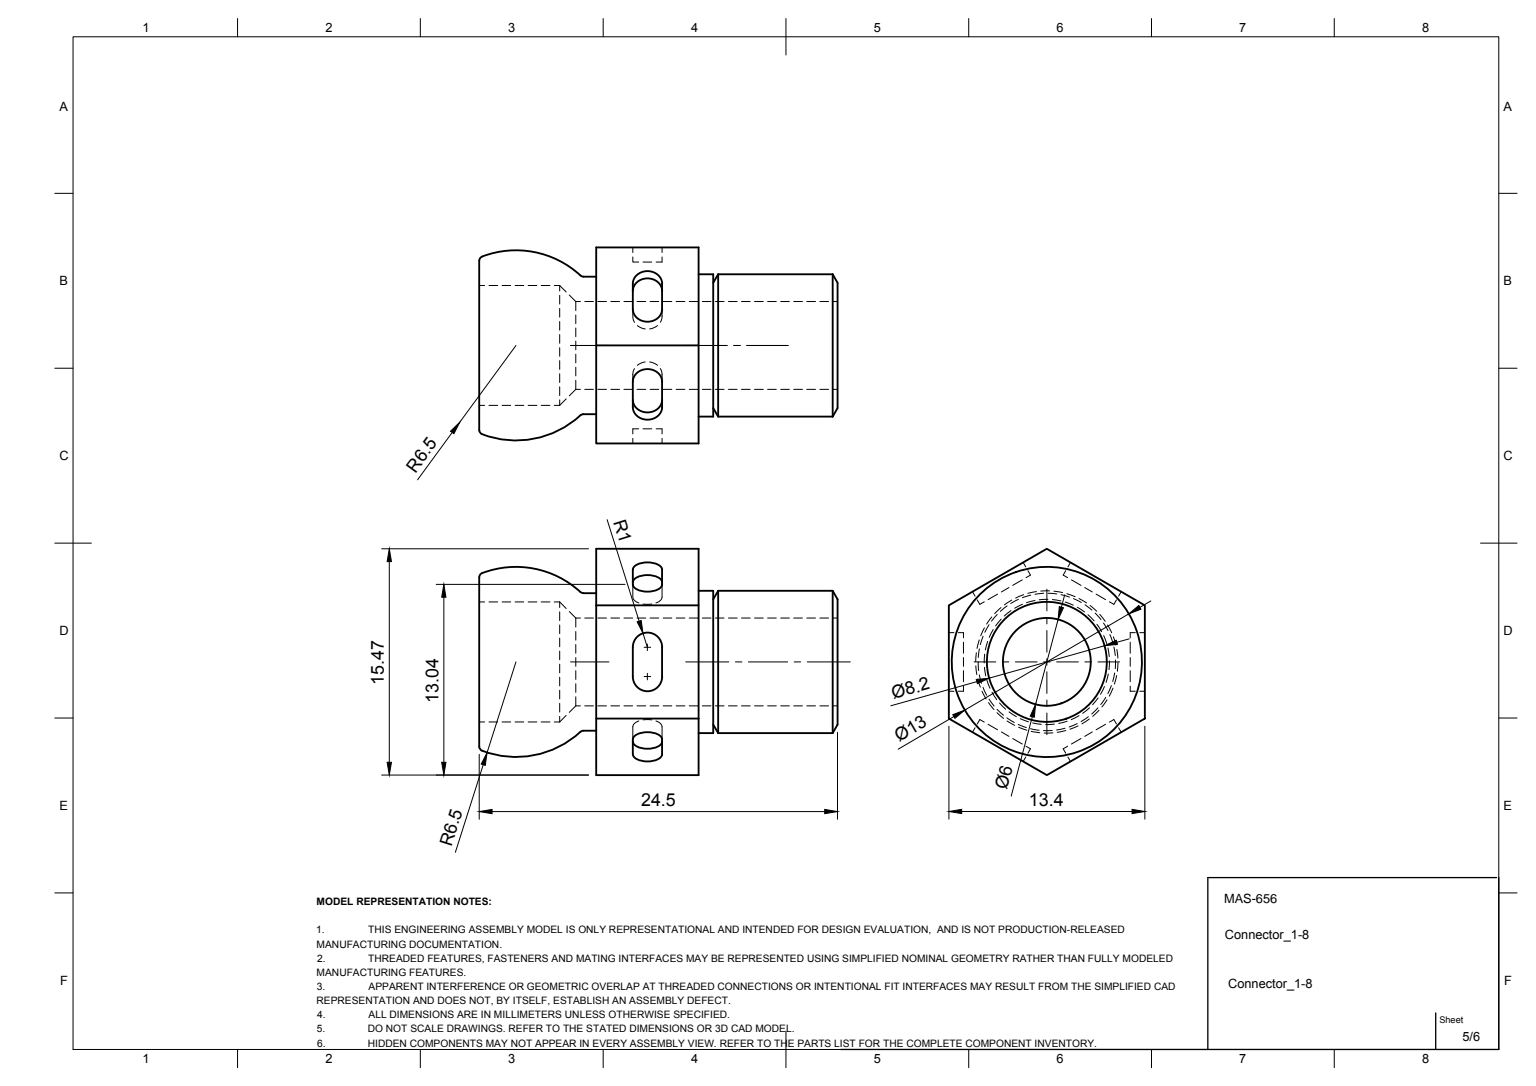
ISO-10303-21;
HEADER;
FILE_DESCRIPTION((''),'2;1');
FILE_NAME('Connector_1-8.step','2026-10-09T09:41:22-07:00',(''),(''),'','','');
FILE_SCHEMA (('AUTOMOTIVE_DESIGN { 1 0 10303 214 3 1 1 }'));
ENDSEC;
DATA;
#10=MECHANICAL_DESIGN_GEOMETRIC_PRESENTATION_REPRESENTATION('',(#74),#4304);
#66=SHAPE_REPRESENTATION_RELATIONSHIP('SRR','None',#4332,#70) ;
#70=ADVANCED_BREP_SHAPE_REPRESENTATION('',(#80),#4301) ;
#74=STYLED_ITEM('',(#4360),#80) ;
#80=MANIFOLD_SOLID_BREP('Body1',#2163) ;
#87=FACE_BOUND('',#638,.T.) ;
#88=FACE_BOUND('',#644,.T.) ;
#89=FACE_BOUND('',#648,.T.) ;
#90=FACE_BOUND('',#650,.T.) ;
#91=FACE_BOUND('',#652,.T.) ;
#92=FACE_BOUND('',#659,.T.) ;
#93=FACE_BOUND('',#661,.T.) ;
#94=FACE_BOUND('',#663,.T.) ;
#95=FACE_BOUND('',#665,.T.) ;
#96=FACE_BOUND('',#667,.T.) ;
#97=FACE_BOUND('',#694,.T.) ;
#119=PLANE('',#2272) ;
#120=PLANE('',#2282) ;
#121=PLANE('',#2288) ;
#122=PLANE('',#2289) ;
#123=PLANE('',#2291) ;
#124=PLANE('',#2296) ;
#125=PLANE('',#2297) ;
#126=PLANE('',#2298) ;
#127=PLANE('',#2301) ;
#128=PLANE('',#2304) ;
#129=PLANE('',#2307) ;
#130=PLANE('',#2310) ;
#131=PLANE('',#2313) ;
#132=PLANE('',#2318) ;
#133=PLANE('',#2319) ;
#134=PLANE('',#2320) ;
#135=PLANE('',#2325) ;
#136=PLANE('',#2326) ;
#137=PLANE('',#2327) ;
#138=PLANE('',#2332) ;
#139=PLANE('',#2333) ;
#140=PLANE('',#2334) ;
#141=PLANE('',#2339) ;
#142=PLANE('',#2340) ;
#143=PLANE('',#2341) ;
#144=PLANE('',#2346) ;
#145=PLANE('',#2347) ;
#146=PLANE('',#2348) ;
#147=PLANE('',#2351) ;
#167=TOROIDAL_SURFACE('',#2353,5.79274121460044,0.300000000000023) ;
#168=TOROIDAL_SURFACE('',#2364,5.00000000000038,0.300000000000023) ;
#181=CYLINDRICAL_SURFACE('',#2274,4.86400000000037) ;
#182=CYLINDRICAL_SURFACE('',#2276,3.00000000000023) ;
#183=CYLINDRICAL_SURFACE('',#2284,4.10000000000031) ;
#184=CYLINDRICAL_SURFACE('',#2286,4.86400000000037) ;
#185=CYLINDRICAL_SURFACE('',#2294,1.00000000000008) ;
#186=CYLINDRICAL_SURFACE('',#2300,1.00000000000008) ;
#187=CYLINDRICAL_SURFACE('',#2316,1.00000000000008) ;
#188=CYLINDRICAL_SURFACE('',#2322,1.00000000000008) ;
#189=CYLINDRICAL_SURFACE('',#2323,1.00000000000008) ;
#190=CYLINDRICAL_SURFACE('',#2329,1.00000000000008) ;
#191=CYLINDRICAL_SURFACE('',#2330,1.00000000000008) ;
#192=CYLINDRICAL_SURFACE('',#2336,1.00000000000008) ;
#193=CYLINDRICAL_SURFACE('',#2337,1.00000000000008) ;
#194=CYLINDRICAL_SURFACE('',#2343,1.00000000000008) ;
#195=CYLINDRICAL_SURFACE('',#2344,1.00000000000008) ;
#196=CYLINDRICAL_SURFACE('',#2350,1.00000000000008) ;
#197=CYLINDRICAL_SURFACE('',#2357,4.70000000000036) ;
#229=LINE('',#3374,#348) ;
#230=LINE('',#3382,#349) ;
#231=LINE('',#3385,#350) ;
#232=LINE('',#3389,#351) ;
#233=LINE('',#3393,#352) ;
#234=LINE('',#3400,#353) ;
#235=LINE('',#3405,#354) ;
#236=LINE('',#3409,#355) ;
#237=LINE('',#3411,#356) ;
#238=LINE('',#3413,#357) ;
#239=LINE('',#3415,#358) ;
#240=LINE('',#3417,#359) ;
#241=LINE('',#3418,#360) ;
#242=LINE('',#3422,#361) ;
#243=LINE('',#3424,#362) ;
#244=LINE('',#3426,#363) ;
#245=LINE('',#3428,#364) ;
#246=LINE('',#3430,#365) ;
#247=LINE('',#3431,#366) ;
#248=LINE('',#3435,#367) ;
#249=LINE('',#3436,#368) ;
#250=LINE('',#3441,#369) ;
#251=LINE('',#3444,#370) ;
#252=LINE('',#3447,#371) ;
#253=LINE('',#3449,#372) ;
#254=LINE('',#3453,#373) ;
#255=LINE('',#3454,#374) ;
#256=LINE('',#3457,#375) ;
#257=LINE('',#3458,#376) ;
#258=LINE('',#3463,#377) ;
#259=LINE('',#3466,#378) ;
#260=LINE('',#3470,#379) ;
#261=LINE('',#3473,#380) ;
#262=LINE('',#3476,#381) ;
#263=LINE('',#3480,#382) ;
#264=LINE('',#3483,#383) ;
#265=LINE('',#3486,#384) ;
#266=LINE('',#3490,#385) ;
#267=LINE('',#3493,#386) ;
#268=LINE('',#3496,#387) ;
#269=LINE('',#3500,#388) ;
#270=LINE('',#3505,#389) ;
#271=LINE('',#3509,#390) ;
#272=LINE('',#3513,#391) ;
#273=LINE('',#3515,#392) ;
#274=LINE('',#3519,#393) ;
#275=LINE('',#3520,#394) ;
#276=LINE('',#3523,#395) ;
#277=LINE('',#3524,#396) ;
#278=LINE('',#3530,#397) ;
#279=LINE('',#3532,#398) ;
#280=LINE('',#3536,#399) ;
#281=LINE('',#3537,#400) ;
#282=LINE('',#3540,#401) ;
#283=LINE('',#3541,#402) ;
#284=LINE('',#3547,#403) ;
#285=LINE('',#3549,#404) ;
#286=LINE('',#3553,#405) ;
#287=LINE('',#3554,#406) ;
#288=LINE('',#3557,#407) ;
#289=LINE('',#3558,#408) ;
#290=LINE('',#3564,#409) ;
#291=LINE('',#3566,#410) ;
#292=LINE('',#3570,#411) ;
#293=LINE('',#3571,#412) ;
#294=LINE('',#3574,#413) ;
#295=LINE('',#3575,#414) ;
#296=LINE('',#3581,#415) ;
#297=LINE('',#3583,#416) ;
#298=LINE('',#3587,#417) ;
#299=LINE('',#3588,#418) ;
#300=LINE('',#3591,#419) ;
#301=LINE('',#3592,#420) ;
#302=LINE('',#3609,#421) ;
#348=VECTOR('',#2652,4.28300000000033) ;
#349=VECTOR('',#2663,4.86400000000037) ;
#350=VECTOR('',#2666,3.00000000000023) ;
#351=VECTOR('',#2671,4.28300000000033) ;
#352=VECTOR('',#2676,3.00000000000023) ;
#353=VECTOR('',#2685,4.10000000000031) ;
#354=VECTOR('',#2692,4.86400000000037) ;
#355=VECTOR('',#2695,1.00000000000008) ;
#356=VECTOR('',#2696,0.999999999999697) ;
#357=VECTOR('',#2697,0.999999999999697) ;
#358=VECTOR('',#2698,1.00000000000008) ;
#359=VECTOR('',#2699,0.999999999999697) ;
#360=VECTOR('',#2700,0.999999999999697) ;
#361=VECTOR('',#2703,0.999999999999697) ;
#362=VECTOR('',#2704,1.00000000000008) ;
#363=VECTOR('',#2705,0.999999999999697) ;
#364=VECTOR('',#2706,0.999999999999697) ;
#365=VECTOR('',#2707,1.00000000000008) ;
#366=VECTOR('',#2708,0.999999999999697) ;
#367=VECTOR('',#2713,1.00000000000008) ;
#368=VECTOR('',#2714,1.00000000000008) ;
#369=VECTOR('',#2717,1.00000000000008) ;
#370=VECTOR('',#2720,1.00000000000008) ;
#371=VECTOR('',#2723,1.00000000000008) ;
#372=VECTOR('',#2724,1.00000000000008) ;
#373=VECTOR('',#2729,1.00000000000008) ;
#374=VECTOR('',#2730,1.00000000000008) ;
#375=VECTOR('',#2733,1.00000000000008) ;
#376=VECTOR('',#2734,1.00000000000008) ;
#377=VECTOR('',#2743,1.00000000000008) ;
#378=VECTOR('',#2744,0.999999999999697) ;
#379=VECTOR('',#2747,0.999999999999697) ;
#380=VECTOR('',#2752,1.00000000000008) ;
#381=VECTOR('',#2753,0.999999999999697) ;
#382=VECTOR('',#2756,0.999999999999697) ;
#383=VECTOR('',#2761,1.00000000000008) ;
#384=VECTOR('',#2762,0.999999999999697) ;
#385=VECTOR('',#2765,0.999999999999697) ;
#386=VECTOR('',#2770,1.00000000000008) ;
#387=VECTOR('',#2771,0.999999999999697) ;
#388=VECTOR('',#2774,0.999999999999697) ;
#389=VECTOR('',#2779,1.00000000000008) ;
#390=VECTOR('',#2782,1.00000000000008) ;
#391=VECTOR('',#2787,1.00000000000008) ;
#392=VECTOR('',#2788,1.00000000000008) ;
#393=VECTOR('',#2793,1.00000000000008) ;
#394=VECTOR('',#2794,1.00000000000008) ;
#395=VECTOR('',#2797,1.00000000000008) ;
#396=VECTOR('',#2798,1.00000000000008) ;
#397=VECTOR('',#2807,0.999999999999697) ;
#398=VECTOR('',#2808,0.999999999999697) ;
#399=VECTOR('',#2813,0.999999999999697) ;
#400=VECTOR('',#2814,0.999999999999697) ;
#401=VECTOR('',#2817,0.999999999999697) ;
#402=VECTOR('',#2818,0.999999999999697) ;
#403=VECTOR('',#2827,0.999999999999697) ;
#404=VECTOR('',#2828,0.999999999999697) ;
#405=VECTOR('',#2833,0.999999999999697) ;
#406=VECTOR('',#2834,0.999999999999697) ;
#407=VECTOR('',#2837,0.999999999999697) ;
#408=VECTOR('',#2838,0.999999999999697) ;
#409=VECTOR('',#2847,0.999999999999696) ;
#410=VECTOR('',#2848,0.999999999999696) ;
#411=VECTOR('',#2853,0.999999999999696) ;
#412=VECTOR('',#2854,0.999999999999697) ;
#413=VECTOR('',#2857,0.999999999999696) ;
#414=VECTOR('',#2858,0.999999999999697) ;
#415=VECTOR('',#2867,0.999999999999696) ;
#416=VECTOR('',#2868,0.999999999999696) ;
#417=VECTOR('',#2873,0.999999999999696) ;
#418=VECTOR('',#2874,0.999999999999697) ;
#419=VECTOR('',#2877,0.999999999999696) ;
#420=VECTOR('',#2878,0.999999999999697) ;
#421=VECTOR('',#2901,4.70000000000036) ;
#463=CONICAL_SURFACE('',#2269,4.28300000000033,1.0471975512) ;
#464=CONICAL_SURFACE('',#2278,4.28300000000033,1.0471975512) ;
#465=CONICAL_SURFACE('',#2280,3.00000000000023,0.785398163397) ;
#498=FACE_OUTER_BOUND('',#636,.T.) ;
#499=FACE_OUTER_BOUND('',#637,.T.) ;
#500=FACE_OUTER_BOUND('',#639,.T.) ;
#501=FACE_OUTER_BOUND('',#640,.T.) ;
#502=FACE_OUTER_BOUND('',#641,.T.) ;
#503=FACE_OUTER_BOUND('',#642,.T.) ;
#504=FACE_OUTER_BOUND('',#643,.T.) ;
#505=FACE_OUTER_BOUND('',#645,.T.) ;
#506=FACE_OUTER_BOUND('',#646,.T.) ;
#507=FACE_OUTER_BOUND('',#647,.T.) ;
#508=FACE_OUTER_BOUND('',#649,.T.) ;
#509=FACE_OUTER_BOUND('',#651,.T.) ;
#510=FACE_OUTER_BOUND('',#653,.T.) ;
#511=FACE_OUTER_BOUND('',#654,.T.) ;
#512=FACE_OUTER_BOUND('',#655,.T.) ;
#513=FACE_OUTER_BOUND('',#656,.T.) ;
#514=FACE_OUTER_BOUND('',#657,.T.) ;
#515=FACE_OUTER_BOUND('',#658,.T.) ;
#516=FACE_OUTER_BOUND('',#660,.T.) ;
#517=FACE_OUTER_BOUND('',#662,.T.) ;
#518=FACE_OUTER_BOUND('',#664,.T.) ;
#519=FACE_OUTER_BOUND('',#666,.T.) ;
#520=FACE_OUTER_BOUND('',#668,.T.) ;
#521=FACE_OUTER_BOUND('',#669,.T.) ;
#522=FACE_OUTER_BOUND('',#670,.T.) ;
#523=FACE_OUTER_BOUND('',#671,.T.) ;
#524=FACE_OUTER_BOUND('',#672,.T.) ;
#525=FACE_OUTER_BOUND('',#673,.T.) ;
#526=FACE_OUTER_BOUND('',#674,.T.) ;
#527=FACE_OUTER_BOUND('',#675,.T.) ;
#528=FACE_OUTER_BOUND('',#676,.T.) ;
#529=FACE_OUTER_BOUND('',#677,.T.) ;
#530=FACE_OUTER_BOUND('',#678,.T.) ;
#531=FACE_OUTER_BOUND('',#679,.T.) ;
#532=FACE_OUTER_BOUND('',#680,.T.) ;
#533=FACE_OUTER_BOUND('',#681,.T.) ;
#534=FACE_OUTER_BOUND('',#682,.T.) ;
#535=FACE_OUTER_BOUND('',#683,.T.) ;
#536=FACE_OUTER_BOUND('',#684,.T.) ;
#537=FACE_OUTER_BOUND('',#685,.T.) ;
#538=FACE_OUTER_BOUND('',#686,.T.) ;
#539=FACE_OUTER_BOUND('',#687,.T.) ;
#540=FACE_OUTER_BOUND('',#688,.T.) ;
#541=FACE_OUTER_BOUND('',#689,.T.) ;
#542=FACE_OUTER_BOUND('',#690,.T.) ;
#543=FACE_OUTER_BOUND('',#691,.T.) ;
#544=FACE_OUTER_BOUND('',#692,.T.) ;
#545=FACE_OUTER_BOUND('',#693,.T.) ;
#546=FACE_OUTER_BOUND('',#695,.T.) ;
#547=FACE_OUTER_BOUND('',#696,.T.) ;
#548=FACE_OUTER_BOUND('',#697,.T.) ;
#549=FACE_OUTER_BOUND('',#698,.T.) ;
#636=EDGE_LOOP('',(#1513,#1514,#1515,#1516)) ;
#637=EDGE_LOOP('',(#1517)) ;
#638=EDGE_LOOP('',(#1518)) ;
#639=EDGE_LOOP('',(#1519,#1520,#1521,#1522)) ;
#640=EDGE_LOOP('',(#1523,#1524,#1525,#1526)) ;
#641=EDGE_LOOP('',(#1527,#1528,#1529,#1530)) ;
#642=EDGE_LOOP('',(#1531,#1532,#1533,#1534)) ;
#643=EDGE_LOOP('',(#1535)) ;
#644=EDGE_LOOP('',(#1536)) ;
#645=EDGE_LOOP('',(#1537,#1538,#1539,#1540)) ;
#646=EDGE_LOOP('',(#1541,#1542,#1543,#1544)) ;
#647=EDGE_LOOP('',(#1545,#1546,#1547,#1548,#1549,#1550)) ;
#648=EDGE_LOOP('',(#1551)) ;
#649=EDGE_LOOP('',(#1552,#1553,#1554,#1555,#1556,#1557)) ;
#650=EDGE_LOOP('',(#1558)) ;
#651=EDGE_LOOP('',(#1559,#1560,#1561,#1562)) ;
#652=EDGE_LOOP('',(#1563,#1564,#1565,#1566)) ;
#653=EDGE_LOOP('',(#1567,#1568,#1569,#1570)) ;
#654=EDGE_LOOP('',(#1571,#1572,#1573,#1574)) ;
#655=EDGE_LOOP('',(#1575,#1576,#1577,#1578)) ;
#656=EDGE_LOOP('',(#1579,#1580,#1581,#1582)) ;
#657=EDGE_LOOP('',(#1583,#1584,#1585,#1586)) ;
#658=EDGE_LOOP('',(#1587,#1588,#1589,#1590)) ;
#659=EDGE_LOOP('',(#1591,#1592,#1593,#1594)) ;
#660=EDGE_LOOP('',(#1595,#1596,#1597,#1598)) ;
#661=EDGE_LOOP('',(#1599,#1600,#1601,#1602)) ;
#662=EDGE_LOOP('',(#1603,#1604,#1605,#1606)) ;
#663=EDGE_LOOP('',(#1607,#1608,#1609,#1610)) ;
#664=EDGE_LOOP('',(#1611,#1612,#1613,#1614)) ;
#665=EDGE_LOOP('',(#1615,#1616,#1617,#1618)) ;
#666=EDGE_LOOP('',(#1619,#1620,#1621,#1622)) ;
#667=EDGE_LOOP('',(#1623,#1624,#1625,#1626)) ;
#668=EDGE_LOOP('',(#1627,#1628,#1629,#1630)) ;
#669=EDGE_LOOP('',(#1631,#1632,#1633,#1634)) ;
#670=EDGE_LOOP('',(#1635,#1636,#1637,#1638)) ;
#671=EDGE_LOOP('',(#1639,#1640,#1641,#1642)) ;
#672=EDGE_LOOP('',(#1643,#1644,#1645,#1646)) ;
#673=EDGE_LOOP('',(#1647,#1648,#1649,#1650)) ;
#674=EDGE_LOOP('',(#1651,#1652,#1653,#1654)) ;
#675=EDGE_LOOP('',(#1655,#1656,#1657,#1658)) ;
#676=EDGE_LOOP('',(#1659,#1660,#1661,#1662)) ;
#677=EDGE_LOOP('',(#1663,#1664,#1665,#1666)) ;
#678=EDGE_LOOP('',(#1667,#1668,#1669,#1670)) ;
#679=EDGE_LOOP('',(#1671,#1672,#1673,#1674)) ;
#680=EDGE_LOOP('',(#1675,#1676,#1677,#1678)) ;
#681=EDGE_LOOP('',(#1679,#1680,#1681,#1682)) ;
#682=EDGE_LOOP('',(#1683,#1684,#1685,#1686)) ;
#683=EDGE_LOOP('',(#1687,#1688,#1689,#1690)) ;
#684=EDGE_LOOP('',(#1691,#1692,#1693,#1694)) ;
#685=EDGE_LOOP('',(#1695,#1696,#1697,#1698)) ;
#686=EDGE_LOOP('',(#1699,#1700,#1701,#1702)) ;
#687=EDGE_LOOP('',(#1703,#1704,#1705,#1706)) ;
#688=EDGE_LOOP('',(#1707,#1708,#1709,#1710)) ;
#689=EDGE_LOOP('',(#1711,#1712,#1713,#1714)) ;
#690=EDGE_LOOP('',(#1715,#1716,#1717,#1718)) ;
#691=EDGE_LOOP('',(#1719,#1720,#1721,#1722)) ;
#692=EDGE_LOOP('',(#1723,#1724,#1725,#1726)) ;
#693=EDGE_LOOP('',(#1727)) ;
#694=EDGE_LOOP('',(#1728)) ;
#695=EDGE_LOOP('',(#1729,#1730,#1731,#1732,#1733)) ;
#696=EDGE_LOOP('',(#1734,#1735,#1736,#1737,#1738)) ;
#697=EDGE_LOOP('',(#1739,#1740,#1741,#1742,#1743,#1744)) ;
#698=EDGE_LOOP('',(#1745,#1746,#1747,#1748,#1749,#1750)) ;
#819=CIRCLE('',#2270,4.86400000000037) ;
#820=CIRCLE('',#2271,4.28300000000033) ;
#821=CIRCLE('',#2273,3.00000000000023) ;
#822=CIRCLE('',#2275,4.86400000000037) ;
#823=CIRCLE('',#2277,3.00000000000023) ;
#824=CIRCLE('',#2279,4.28300000000033) ;
#825=CIRCLE('',#2281,4.10000000000031) ;
#826=CIRCLE('',#2283,4.86400000000037) ;
#827=CIRCLE('',#2285,4.10000000000031) ;
#828=CIRCLE('',#2287,4.86400000000037) ;
#829=CIRCLE('',#2290,4.70000000000036) ;
#830=CIRCLE('',#2292,1.00000000000008) ;
#831=CIRCLE('',#2293,1.00000000000008) ;
#832=CIRCLE('',#2295,1.00000000000008) ;
#833=CIRCLE('',#2299,1.00000000000008) ;
#834=CIRCLE('',#2302,1.00000000000008) ;
#835=CIRCLE('',#2303,1.00000000000008) ;
#836=CIRCLE('',#2305,1.00000000000008) ;
#837=CIRCLE('',#2306,1.00000000000008) ;
#838=CIRCLE('',#2308,1.00000000000008) ;
#839=CIRCLE('',#2309,1.00000000000008) ;
#840=CIRCLE('',#2311,1.00000000000008) ;
#841=CIRCLE('',#2312,1.00000000000008) ;
#842=CIRCLE('',#2314,1.00000000000008) ;
#843=CIRCLE('',#2315,1.00000000000008) ;
#844=CIRCLE('',#2317,1.00000000000008) ;
#845=CIRCLE('',#2321,1.00000000000008) ;
#846=CIRCLE('',#2324,1.00000000000008) ;
#847=CIRCLE('',#2328,1.00000000000008) ;
#848=CIRCLE('',#2331,1.00000000000008) ;
#849=CIRCLE('',#2335,1.00000000000008) ;
#850=CIRCLE('',#2338,1.00000000000008) ;
#851=CIRCLE('',#2342,1.00000000000008) ;
#852=CIRCLE('',#2345,1.00000000000008) ;
#853=CIRCLE('',#2349,1.00000000000008) ;
#854=CIRCLE('',#2352,5.79274121460045) ;
#855=CIRCLE('',#2354,0.300000000000023) ;
#856=CIRCLE('',#2355,6.07303514434047) ;
#857=CIRCLE('',#2356,6.07303514434047) ;
#858=CIRCLE('',#2358,4.70000000000036) ;
#859=CIRCLE('',#2359,4.70000000000036) ;
#860=CIRCLE('',#2361,6.50000000000051) ;
#861=CIRCLE('',#2362,4.77941176471037) ;
#862=CIRCLE('',#2363,4.77941176471037) ;
#863=CIRCLE('',#2365,0.300000000000023) ;
#978=VERTEX_POINT('',#3371) ;
#979=VERTEX_POINT('',#3373) ;
#980=VERTEX_POINT('',#3377) ;
#981=VERTEX_POINT('',#3380) ;
#982=VERTEX_POINT('',#3384) ;
#983=VERTEX_POINT('',#3388) ;
#984=VERTEX_POINT('',#3392) ;
#985=VERTEX_POINT('',#3396) ;
#986=VERTEX_POINT('',#3399) ;
#987=VERTEX_POINT('',#3403) ;
#988=VERTEX_POINT('',#3407) ;
#989=VERTEX_POINT('',#3408) ;
#990=VERTEX_POINT('',#3410) ;
#991=VERTEX_POINT('',#3412) ;
#992=VERTEX_POINT('',#3414) ;
#993=VERTEX_POINT('',#3416) ;
#994=VERTEX_POINT('',#3420) ;
#995=VERTEX_POINT('',#3421) ;
#996=VERTEX_POINT('',#3423) ;
#997=VERTEX_POINT('',#3425) ;
#998=VERTEX_POINT('',#3427) ;
#999=VERTEX_POINT('',#3429) ;
#1000=VERTEX_POINT('',#3432) ;
#1001=VERTEX_POINT('',#3437) ;
#1002=VERTEX_POINT('',#3438) ;
#1003=VERTEX_POINT('',#3440) ;
#1004=VERTEX_POINT('',#3442) ;
#1005=VERTEX_POINT('',#3446) ;
#1006=VERTEX_POINT('',#3448) ;
#1007=VERTEX_POINT('',#3452) ;
#1008=VERTEX_POINT('',#3456) ;
#1009=VERTEX_POINT('',#3464) ;
#1010=VERTEX_POINT('',#3465) ;
#1011=VERTEX_POINT('',#3467) ;
#1012=VERTEX_POINT('',#3469) ;
#1013=VERTEX_POINT('',#3474) ;
#1014=VERTEX_POINT('',#3475) ;
#1015=VERTEX_POINT('',#3477) ;
#1016=VERTEX_POINT('',#3479) ;
#1017=VERTEX_POINT('',#3484) ;
#1018=VERTEX_POINT('',#3485) ;
#1019=VERTEX_POINT('',#3487) ;
#1020=VERTEX_POINT('',#3489) ;
#1021=VERTEX_POINT('',#3494) ;
#1022=VERTEX_POINT('',#3495) ;
#1023=VERTEX_POINT('',#3497) ;
#1024=VERTEX_POINT('',#3499) ;
#1025=VERTEX_POINT('',#3503) ;
#1026=VERTEX_POINT('',#3504) ;
#1027=VERTEX_POINT('',#3506) ;
#1028=VERTEX_POINT('',#3508) ;
#1029=VERTEX_POINT('',#3512) ;
#1030=VERTEX_POINT('',#3514) ;
#1031=VERTEX_POINT('',#3518) ;
#1032=VERTEX_POINT('',#3522) ;
#1033=VERTEX_POINT('',#3529) ;
#1034=VERTEX_POINT('',#3531) ;
#1035=VERTEX_POINT('',#3535) ;
#1036=VERTEX_POINT('',#3539) ;
#1037=VERTEX_POINT('',#3546) ;
#1038=VERTEX_POINT('',#3548) ;
#1039=VERTEX_POINT('',#3552) ;
#1040=VERTEX_POINT('',#3556) ;
#1041=VERTEX_POINT('',#3563) ;
#1042=VERTEX_POINT('',#3565) ;
#1043=VERTEX_POINT('',#3569) ;
#1044=VERTEX_POINT('',#3573) ;
#1045=VERTEX_POINT('',#3580) ;
#1046=VERTEX_POINT('',#3582) ;
#1047=VERTEX_POINT('',#3586) ;
#1048=VERTEX_POINT('',#3590) ;
#1049=VERTEX_POINT('',#3597) ;
#1050=VERTEX_POINT('',#3600) ;
#1051=VERTEX_POINT('',#3602) ;
#1052=VERTEX_POINT('',#3606) ;
#1053=VERTEX_POINT('',#3607) ;
#1054=VERTEX_POINT('',#3612) ;
#1055=VERTEX_POINT('',#3614) ;
#1178=EDGE_CURVE('',#978,#978,#819,.T.) ;
#1179=EDGE_CURVE('',#978,#979,#229,.T.) ;
#1180=EDGE_CURVE('',#979,#979,#820,.T.) ;
#1181=EDGE_CURVE('',#980,#980,#821,.T.) ;
#1182=EDGE_CURVE('',#981,#981,#822,.T.) ;
#1183=EDGE_CURVE('',#981,#978,#230,.T.) ;
#1184=EDGE_CURVE('',#980,#982,#231,.T.) ;
#1185=EDGE_CURVE('',#982,#982,#823,.T.) ;
#1186=EDGE_CURVE('',#981,#983,#232,.T.) ;
#1187=EDGE_CURVE('',#983,#983,#824,.F.) ;
#1188=EDGE_CURVE('',#982,#984,#233,.T.) ;
#1189=EDGE_CURVE('',#984,#984,#825,.T.) ;
#1190=EDGE_CURVE('',#985,#985,#826,.T.) ;
#1191=EDGE_CURVE('',#984,#986,#234,.T.) ;
#1192=EDGE_CURVE('',#986,#986,#827,.T.) ;
#1193=EDGE_CURVE('',#987,#987,#828,.T.) ;
#1194=EDGE_CURVE('',#987,#985,#235,.T.) ;
#1195=EDGE_CURVE('',#988,#989,#236,.T.) ;
#1196=EDGE_CURVE('',#989,#990,#237,.T.) ;
#1197=EDGE_CURVE('',#990,#991,#238,.T.) ;
#1198=EDGE_CURVE('',#991,#992,#239,.T.) ;
#1199=EDGE_CURVE('',#992,#993,#240,.T.) ;
#1200=EDGE_CURVE('',#993,#988,#241,.T.) ;
#1201=EDGE_CURVE('',#994,#995,#242,.T.) ;
#1202=EDGE_CURVE('',#996,#994,#243,.T.) ;
#1203=EDGE_CURVE('',#997,#996,#244,.T.) ;
#1204=EDGE_CURVE('',#998,#997,#245,.T.) ;
#1205=EDGE_CURVE('',#999,#998,#246,.T.) ;
#1206=EDGE_CURVE('',#995,#999,#247,.T.) ;
#1207=EDGE_CURVE('',#1000,#1000,#829,.T.) ;
#1208=EDGE_CURVE('',#992,#994,#248,.T.) ;
#1209=EDGE_CURVE('',#991,#996,#249,.T.) ;
#1210=EDGE_CURVE('',#1001,#1002,#830,.F.) ;
#1211=EDGE_CURVE('',#1003,#1001,#250,.F.) ;
#1212=EDGE_CURVE('',#1004,#1003,#831,.F.) ;
#1213=EDGE_CURVE('',#1002,#1004,#251,.F.) ;
#1214=EDGE_CURVE('',#1004,#1005,#252,.F.) ;
#1215=EDGE_CURVE('',#1003,#1006,#253,.F.) ;
#1216=EDGE_CURVE('',#1005,#1006,#832,.T.) ;
#1217=EDGE_CURVE('',#1002,#1007,#254,.T.) ;
#1218=EDGE_CURVE('',#1007,#1005,#255,.F.) ;
#1219=EDGE_CURVE('',#1001,#1008,#256,.T.) ;
#1220=EDGE_CURVE('',#1006,#1008,#257,.F.) ;
#1221=EDGE_CURVE('',#1008,#1007,#833,.T.) ;
#1222=EDGE_CURVE('',#990,#997,#258,.T.) ;
#1223=EDGE_CURVE('',#1009,#1010,#259,.F.) ;
#1224=EDGE_CURVE('',#1011,#1009,#834,.F.) ;
#1225=EDGE_CURVE('',#1012,#1011,#260,.F.) ;
#1226=EDGE_CURVE('',#1010,#1012,#835,.F.) ;
#1227=EDGE_CURVE('',#993,#995,#261,.T.) ;
#1228=EDGE_CURVE('',#1013,#1014,#262,.F.) ;
#1229=EDGE_CURVE('',#1015,#1013,#836,.F.) ;
#1230=EDGE_CURVE('',#1016,#1015,#263,.F.) ;
#1231=EDGE_CURVE('',#1014,#1016,#837,.F.) ;
#1232=EDGE_CURVE('',#989,#998,#264,.T.) ;
#1233=EDGE_CURVE('',#1017,#1018,#265,.F.) ;
#1234=EDGE_CURVE('',#1019,#1017,#838,.F.) ;
#1235=EDGE_CURVE('',#1020,#1019,#266,.F.) ;
#1236=EDGE_CURVE('',#1018,#1020,#839,.F.) ;
#1237=EDGE_CURVE('',#988,#999,#267,.T.) ;
#1238=EDGE_CURVE('',#1021,#1022,#268,.F.) ;
#1239=EDGE_CURVE('',#1023,#1021,#840,.F.) ;
#1240=EDGE_CURVE('',#1024,#1023,#269,.F.) ;
#1241=EDGE_CURVE('',#1022,#1024,#841,.F.) ;
#1242=EDGE_CURVE('',#1025,#1026,#270,.F.) ;
#1243=EDGE_CURVE('',#1027,#1025,#842,.F.) ;
#1244=EDGE_CURVE('',#1028,#1027,#271,.F.) ;
#1245=EDGE_CURVE('',#1026,#1028,#843,.F.) ;
#1246=EDGE_CURVE('',#1027,#1029,#272,.F.) ;
#1247=EDGE_CURVE('',#1025,#1030,#273,.F.) ;
#1248=EDGE_CURVE('',#1029,#1030,#844,.T.) ;
#1249=EDGE_CURVE('',#1028,#1031,#274,.T.) ;
#1250=EDGE_CURVE('',#1031,#1029,#275,.F.) ;
#1251=EDGE_CURVE('',#1026,#1032,#276,.T.) ;
#1252=EDGE_CURVE('',#1030,#1032,#277,.F.) ;
#1253=EDGE_CURVE('',#1032,#1031,#845,.T.) ;
#1254=EDGE_CURVE('',#1015,#1033,#278,.F.) ;
#1255=EDGE_CURVE('',#1013,#1034,#279,.F.) ;
#1256=EDGE_CURVE('',#1033,#1034,#846,.T.) ;
#1257=EDGE_CURVE('',#1016,#1035,#280,.T.) ;
#1258=EDGE_CURVE('',#1035,#1033,#281,.F.) ;
#1259=EDGE_CURVE('',#1014,#1036,#282,.T.) ;
#1260=EDGE_CURVE('',#1034,#1036,#283,.F.) ;
#1261=EDGE_CURVE('',#1036,#1035,#847,.T.) ;
#1262=EDGE_CURVE('',#1019,#1037,#284,.F.) ;
#1263=EDGE_CURVE('',#1017,#1038,#285,.F.) ;
#1264=EDGE_CURVE('',#1037,#1038,#848,.T.) ;
#1265=EDGE_CURVE('',#1020,#1039,#286,.T.) ;
#1266=EDGE_CURVE('',#1039,#1037,#287,.F.) ;
#1267=EDGE_CURVE('',#1018,#1040,#288,.T.) ;
#1268=EDGE_CURVE('',#1038,#1040,#289,.F.) ;
#1269=EDGE_CURVE('',#1040,#1039,#849,.T.) ;
#1270=EDGE_CURVE('',#1011,#1041,#290,.F.) ;
#1271=EDGE_CURVE('',#1009,#1042,#291,.F.) ;
#1272=EDGE_CURVE('',#1041,#1042,#850,.T.) ;
#1273=EDGE_CURVE('',#1012,#1043,#292,.T.) ;
#1274=EDGE_CURVE('',#1043,#1041,#293,.F.) ;
#1275=EDGE_CURVE('',#1010,#1044,#294,.T.) ;
#1276=EDGE_CURVE('',#1042,#1044,#295,.F.) ;
#1277=EDGE_CURVE('',#1044,#1043,#851,.T.) ;
#1278=EDGE_CURVE('',#1023,#1045,#296,.F.) ;
#1279=EDGE_CURVE('',#1021,#1046,#297,.F.) ;
#1280=EDGE_CURVE('',#1045,#1046,#852,.T.) ;
#1281=EDGE_CURVE('',#1024,#1047,#298,.T.) ;
#1282=EDGE_CURVE('',#1047,#1045,#299,.F.) ;
#1283=EDGE_CURVE('',#1022,#1048,#300,.T.) ;
#1284=EDGE_CURVE('',#1046,#1048,#301,.F.) ;
#1285=EDGE_CURVE('',#1048,#1047,#853,.T.) ;
#1286=EDGE_CURVE('',#1049,#1049,#854,.T.) ;
#1287=EDGE_CURVE('',#1049,#1050,#855,.T.) ;
#1288=EDGE_CURVE('',#1050,#1051,#856,.T.) ;
#1289=EDGE_CURVE('',#1051,#1050,#857,.T.) ;
#1290=EDGE_CURVE('',#1052,#1053,#858,.F.) ;
#1291=EDGE_CURVE('',#1053,#1000,#302,.T.) ;
#1292=EDGE_CURVE('',#1053,#1052,#859,.F.) ;
#1293=EDGE_CURVE('',#1051,#1054,#860,.T.) ;
#1294=EDGE_CURVE('',#1055,#1054,#861,.F.) ;
#1295=EDGE_CURVE('',#1054,#1055,#862,.F.) ;
#1296=EDGE_CURVE('',#1055,#1052,#863,.T.) ;
#1513=ORIENTED_EDGE('',*,*,#1178,.F.) ;
#1514=ORIENTED_EDGE('',*,*,#1179,.T.) ;
#1515=ORIENTED_EDGE('',*,*,#1180,.T.) ;
#1516=ORIENTED_EDGE('',*,*,#1179,.F.) ;
#1517=ORIENTED_EDGE('',*,*,#1180,.F.) ;
#1518=ORIENTED_EDGE('',*,*,#1181,.T.) ;
#1519=ORIENTED_EDGE('',*,*,#1182,.F.) ;
#1520=ORIENTED_EDGE('',*,*,#1183,.T.) ;
#1521=ORIENTED_EDGE('',*,*,#1178,.T.) ;
#1522=ORIENTED_EDGE('',*,*,#1183,.F.) ;
#1523=ORIENTED_EDGE('',*,*,#1181,.F.) ;
#1524=ORIENTED_EDGE('',*,*,#1184,.T.) ;
#1525=ORIENTED_EDGE('',*,*,#1185,.T.) ;
#1526=ORIENTED_EDGE('',*,*,#1184,.F.) ;
#1527=ORIENTED_EDGE('',*,*,#1182,.T.) ;
#1528=ORIENTED_EDGE('',*,*,#1186,.T.) ;
#1529=ORIENTED_EDGE('',*,*,#1187,.F.) ;
#1530=ORIENTED_EDGE('',*,*,#1186,.F.) ;
#1531=ORIENTED_EDGE('',*,*,#1185,.F.) ;
#1532=ORIENTED_EDGE('',*,*,#1188,.T.) ;
#1533=ORIENTED_EDGE('',*,*,#1189,.T.) ;
#1534=ORIENTED_EDGE('',*,*,#1188,.F.) ;
#1535=ORIENTED_EDGE('',*,*,#1190,.F.) ;
#1536=ORIENTED_EDGE('',*,*,#1187,.T.) ;
#1537=ORIENTED_EDGE('',*,*,#1189,.F.) ;
#1538=ORIENTED_EDGE('',*,*,#1191,.T.) ;
#1539=ORIENTED_EDGE('',*,*,#1192,.T.) ;
#1540=ORIENTED_EDGE('',*,*,#1191,.F.) ;
#1541=ORIENTED_EDGE('',*,*,#1193,.F.) ;
#1542=ORIENTED_EDGE('',*,*,#1194,.T.) ;
#1543=ORIENTED_EDGE('',*,*,#1190,.T.) ;
#1544=ORIENTED_EDGE('',*,*,#1194,.F.) ;
#1545=ORIENTED_EDGE('',*,*,#1195,.T.) ;
#1546=ORIENTED_EDGE('',*,*,#1196,.T.) ;
#1547=ORIENTED_EDGE('',*,*,#1197,.T.) ;
#1548=ORIENTED_EDGE('',*,*,#1198,.T.) ;
#1549=ORIENTED_EDGE('',*,*,#1199,.T.) ;
#1550=ORIENTED_EDGE('',*,*,#1200,.T.) ;
#1551=ORIENTED_EDGE('',*,*,#1193,.T.) ;
#1552=ORIENTED_EDGE('',*,*,#1201,.F.) ;
#1553=ORIENTED_EDGE('',*,*,#1202,.F.) ;
#1554=ORIENTED_EDGE('',*,*,#1203,.F.) ;
#1555=ORIENTED_EDGE('',*,*,#1204,.F.) ;
#1556=ORIENTED_EDGE('',*,*,#1205,.F.) ;
#1557=ORIENTED_EDGE('',*,*,#1206,.F.) ;
#1558=ORIENTED_EDGE('',*,*,#1207,.F.) ;
#1559=ORIENTED_EDGE('',*,*,#1202,.T.) ;
#1560=ORIENTED_EDGE('',*,*,#1208,.F.) ;
#1561=ORIENTED_EDGE('',*,*,#1198,.F.) ;
#1562=ORIENTED_EDGE('',*,*,#1209,.T.) ;
#1563=ORIENTED_EDGE('',*,*,#1210,.F.) ;
#1564=ORIENTED_EDGE('',*,*,#1211,.F.) ;
#1565=ORIENTED_EDGE('',*,*,#1212,.F.) ;
#1566=ORIENTED_EDGE('',*,*,#1213,.F.) ;
#1567=ORIENTED_EDGE('',*,*,#1214,.F.) ;
#1568=ORIENTED_EDGE('',*,*,#1212,.T.) ;
#1569=ORIENTED_EDGE('',*,*,#1215,.T.) ;
#1570=ORIENTED_EDGE('',*,*,#1216,.F.) ;
#1571=ORIENTED_EDGE('',*,*,#1217,.F.) ;
#1572=ORIENTED_EDGE('',*,*,#1213,.T.) ;
#1573=ORIENTED_EDGE('',*,*,#1214,.T.) ;
#1574=ORIENTED_EDGE('',*,*,#1218,.F.) ;
#1575=ORIENTED_EDGE('',*,*,#1215,.F.) ;
#1576=ORIENTED_EDGE('',*,*,#1211,.T.) ;
#1577=ORIENTED_EDGE('',*,*,#1219,.T.) ;
#1578=ORIENTED_EDGE('',*,*,#1220,.F.) ;
#1579=ORIENTED_EDGE('',*,*,#1216,.T.) ;
#1580=ORIENTED_EDGE('',*,*,#1220,.T.) ;
#1581=ORIENTED_EDGE('',*,*,#1221,.T.) ;
#1582=ORIENTED_EDGE('',*,*,#1218,.T.) ;
#1583=ORIENTED_EDGE('',*,*,#1219,.F.) ;
#1584=ORIENTED_EDGE('',*,*,#1210,.T.) ;
#1585=ORIENTED_EDGE('',*,*,#1217,.T.) ;
#1586=ORIENTED_EDGE('',*,*,#1221,.F.) ;
#1587=ORIENTED_EDGE('',*,*,#1203,.T.) ;
#1588=ORIENTED_EDGE('',*,*,#1209,.F.) ;
#1589=ORIENTED_EDGE('',*,*,#1197,.F.) ;
#1590=ORIENTED_EDGE('',*,*,#1222,.T.) ;
#1591=ORIENTED_EDGE('',*,*,#1223,.F.) ;
#1592=ORIENTED_EDGE('',*,*,#1224,.F.) ;
#1593=ORIENTED_EDGE('',*,*,#1225,.F.) ;
#1594=ORIENTED_EDGE('',*,*,#1226,.F.) ;
#1595=ORIENTED_EDGE('',*,*,#1201,.T.) ;
#1596=ORIENTED_EDGE('',*,*,#1227,.F.) ;
#1597=ORIENTED_EDGE('',*,*,#1199,.F.) ;
#1598=ORIENTED_EDGE('',*,*,#1208,.T.) ;
#1599=ORIENTED_EDGE('',*,*,#1228,.F.) ;
#1600=ORIENTED_EDGE('',*,*,#1229,.F.) ;
#1601=ORIENTED_EDGE('',*,*,#1230,.F.) ;
#1602=ORIENTED_EDGE('',*,*,#1231,.F.) ;
#1603=ORIENTED_EDGE('',*,*,#1204,.T.) ;
#1604=ORIENTED_EDGE('',*,*,#1222,.F.) ;
#1605=ORIENTED_EDGE('',*,*,#1196,.F.) ;
#1606=ORIENTED_EDGE('',*,*,#1232,.T.) ;
#1607=ORIENTED_EDGE('',*,*,#1233,.F.) ;
#1608=ORIENTED_EDGE('',*,*,#1234,.F.) ;
#1609=ORIENTED_EDGE('',*,*,#1235,.F.) ;
#1610=ORIENTED_EDGE('',*,*,#1236,.F.) ;
#1611=ORIENTED_EDGE('',*,*,#1206,.T.) ;
#1612=ORIENTED_EDGE('',*,*,#1237,.F.) ;
#1613=ORIENTED_EDGE('',*,*,#1200,.F.) ;
#1614=ORIENTED_EDGE('',*,*,#1227,.T.) ;
#1615=ORIENTED_EDGE('',*,*,#1238,.F.) ;
#1616=ORIENTED_EDGE('',*,*,#1239,.F.) ;
#1617=ORIENTED_EDGE('',*,*,#1240,.F.) ;
#1618=ORIENTED_EDGE('',*,*,#1241,.F.) ;
#1619=ORIENTED_EDGE('',*,*,#1205,.T.) ;
#1620=ORIENTED_EDGE('',*,*,#1232,.F.) ;
#1621=ORIENTED_EDGE('',*,*,#1195,.F.) ;
#1622=ORIENTED_EDGE('',*,*,#1237,.T.) ;
#1623=ORIENTED_EDGE('',*,*,#1242,.F.) ;
#1624=ORIENTED_EDGE('',*,*,#1243,.F.) ;
#1625=ORIENTED_EDGE('',*,*,#1244,.F.) ;
#1626=ORIENTED_EDGE('',*,*,#1245,.F.) ;
#1627=ORIENTED_EDGE('',*,*,#1246,.F.) ;
#1628=ORIENTED_EDGE('',*,*,#1243,.T.) ;
#1629=ORIENTED_EDGE('',*,*,#1247,.T.) ;
#1630=ORIENTED_EDGE('',*,*,#1248,.F.) ;
#1631=ORIENTED_EDGE('',*,*,#1249,.F.) ;
#1632=ORIENTED_EDGE('',*,*,#1244,.T.) ;
#1633=ORIENTED_EDGE('',*,*,#1246,.T.) ;
#1634=ORIENTED_EDGE('',*,*,#1250,.F.) ;
#1635=ORIENTED_EDGE('',*,*,#1247,.F.) ;
#1636=ORIENTED_EDGE('',*,*,#1242,.T.) ;
#1637=ORIENTED_EDGE('',*,*,#1251,.T.) ;
#1638=ORIENTED_EDGE('',*,*,#1252,.F.) ;
#1639=ORIENTED_EDGE('',*,*,#1248,.T.) ;
#1640=ORIENTED_EDGE('',*,*,#1252,.T.) ;
#1641=ORIENTED_EDGE('',*,*,#1253,.T.) ;
#1642=ORIENTED_EDGE('',*,*,#1250,.T.) ;
#1643=ORIENTED_EDGE('',*,*,#1251,.F.) ;
#1644=ORIENTED_EDGE('',*,*,#1245,.T.) ;
#1645=ORIENTED_EDGE('',*,*,#1249,.T.) ;
#1646=ORIENTED_EDGE('',*,*,#1253,.F.) ;
#1647=ORIENTED_EDGE('',*,*,#1254,.F.) ;
#1648=ORIENTED_EDGE('',*,*,#1229,.T.) ;
#1649=ORIENTED_EDGE('',*,*,#1255,.T.) ;
#1650=ORIENTED_EDGE('',*,*,#1256,.F.) ;
#1651=ORIENTED_EDGE('',*,*,#1257,.F.) ;
#1652=ORIENTED_EDGE('',*,*,#1230,.T.) ;
#1653=ORIENTED_EDGE('',*,*,#1254,.T.) ;
#1654=ORIENTED_EDGE('',*,*,#1258,.F.) ;
#1655=ORIENTED_EDGE('',*,*,#1255,.F.) ;
#1656=ORIENTED_EDGE('',*,*,#1228,.T.) ;
#1657=ORIENTED_EDGE('',*,*,#1259,.T.) ;
#1658=ORIENTED_EDGE('',*,*,#1260,.F.) ;
#1659=ORIENTED_EDGE('',*,*,#1256,.T.) ;
#1660=ORIENTED_EDGE('',*,*,#1260,.T.) ;
#1661=ORIENTED_EDGE('',*,*,#1261,.T.) ;
#1662=ORIENTED_EDGE('',*,*,#1258,.T.) ;
#1663=ORIENTED_EDGE('',*,*,#1259,.F.) ;
#1664=ORIENTED_EDGE('',*,*,#1231,.T.) ;
#1665=ORIENTED_EDGE('',*,*,#1257,.T.) ;
#1666=ORIENTED_EDGE('',*,*,#1261,.F.) ;
#1667=ORIENTED_EDGE('',*,*,#1262,.F.) ;
#1668=ORIENTED_EDGE('',*,*,#1234,.T.) ;
#1669=ORIENTED_EDGE('',*,*,#1263,.T.) ;
#1670=ORIENTED_EDGE('',*,*,#1264,.F.) ;
#1671=ORIENTED_EDGE('',*,*,#1265,.F.) ;
#1672=ORIENTED_EDGE('',*,*,#1235,.T.) ;
#1673=ORIENTED_EDGE('',*,*,#1262,.T.) ;
#1674=ORIENTED_EDGE('',*,*,#1266,.F.) ;
#1675=ORIENTED_EDGE('',*,*,#1263,.F.) ;
#1676=ORIENTED_EDGE('',*,*,#1233,.T.) ;
#1677=ORIENTED_EDGE('',*,*,#1267,.T.) ;
#1678=ORIENTED_EDGE('',*,*,#1268,.F.) ;
#1679=ORIENTED_EDGE('',*,*,#1264,.T.) ;
#1680=ORIENTED_EDGE('',*,*,#1268,.T.) ;
#1681=ORIENTED_EDGE('',*,*,#1269,.T.) ;
#1682=ORIENTED_EDGE('',*,*,#1266,.T.) ;
#1683=ORIENTED_EDGE('',*,*,#1267,.F.) ;
#1684=ORIENTED_EDGE('',*,*,#1236,.T.) ;
#1685=ORIENTED_EDGE('',*,*,#1265,.T.) ;
#1686=ORIENTED_EDGE('',*,*,#1269,.F.) ;
#1687=ORIENTED_EDGE('',*,*,#1270,.F.) ;
#1688=ORIENTED_EDGE('',*,*,#1224,.T.) ;
#1689=ORIENTED_EDGE('',*,*,#1271,.T.) ;
#1690=ORIENTED_EDGE('',*,*,#1272,.F.) ;
#1691=ORIENTED_EDGE('',*,*,#1273,.F.) ;
#1692=ORIENTED_EDGE('',*,*,#1225,.T.) ;
#1693=ORIENTED_EDGE('',*,*,#1270,.T.) ;
#1694=ORIENTED_EDGE('',*,*,#1274,.F.) ;
#1695=ORIENTED_EDGE('',*,*,#1271,.F.) ;
#1696=ORIENTED_EDGE('',*,*,#1223,.T.) ;
#1697=ORIENTED_EDGE('',*,*,#1275,.T.) ;
#1698=ORIENTED_EDGE('',*,*,#1276,.F.) ;
#1699=ORIENTED_EDGE('',*,*,#1272,.T.) ;
#1700=ORIENTED_EDGE('',*,*,#1276,.T.) ;
#1701=ORIENTED_EDGE('',*,*,#1277,.T.) ;
#1702=ORIENTED_EDGE('',*,*,#1274,.T.) ;
#1703=ORIENTED_EDGE('',*,*,#1275,.F.) ;
#1704=ORIENTED_EDGE('',*,*,#1226,.T.) ;
#1705=ORIENTED_EDGE('',*,*,#1273,.T.) ;
#1706=ORIENTED_EDGE('',*,*,#1277,.F.) ;
#1707=ORIENTED_EDGE('',*,*,#1278,.F.) ;
#1708=ORIENTED_EDGE('',*,*,#1239,.T.) ;
#1709=ORIENTED_EDGE('',*,*,#1279,.T.) ;
#1710=ORIENTED_EDGE('',*,*,#1280,.F.) ;
#1711=ORIENTED_EDGE('',*,*,#1281,.F.) ;
#1712=ORIENTED_EDGE('',*,*,#1240,.T.) ;
#1713=ORIENTED_EDGE('',*,*,#1278,.T.) ;
#1714=ORIENTED_EDGE('',*,*,#1282,.F.) ;
#1715=ORIENTED_EDGE('',*,*,#1279,.F.) ;
#1716=ORIENTED_EDGE('',*,*,#1238,.T.) ;
#1717=ORIENTED_EDGE('',*,*,#1283,.T.) ;
#1718=ORIENTED_EDGE('',*,*,#1284,.F.) ;
#1719=ORIENTED_EDGE('',*,*,#1280,.T.) ;
#1720=ORIENTED_EDGE('',*,*,#1284,.T.) ;
#1721=ORIENTED_EDGE('',*,*,#1285,.T.) ;
#1722=ORIENTED_EDGE('',*,*,#1282,.T.) ;
#1723=ORIENTED_EDGE('',*,*,#1283,.F.) ;
#1724=ORIENTED_EDGE('',*,*,#1241,.T.) ;
#1725=ORIENTED_EDGE('',*,*,#1281,.T.) ;
#1726=ORIENTED_EDGE('',*,*,#1285,.F.) ;
#1727=ORIENTED_EDGE('',*,*,#1286,.T.) ;
#1728=ORIENTED_EDGE('',*,*,#1192,.F.) ;
#1729=ORIENTED_EDGE('',*,*,#1286,.F.) ;
#1730=ORIENTED_EDGE('',*,*,#1287,.T.) ;
#1731=ORIENTED_EDGE('',*,*,#1288,.T.) ;
#1732=ORIENTED_EDGE('',*,*,#1289,.T.) ;
#1733=ORIENTED_EDGE('',*,*,#1287,.F.) ;
#1734=ORIENTED_EDGE('',*,*,#1290,.T.) ;
#1735=ORIENTED_EDGE('',*,*,#1291,.T.) ;
#1736=ORIENTED_EDGE('',*,*,#1207,.T.) ;
#1737=ORIENTED_EDGE('',*,*,#1291,.F.) ;
#1738=ORIENTED_EDGE('',*,*,#1292,.T.) ;
#1739=ORIENTED_EDGE('',*,*,#1289,.F.) ;
#1740=ORIENTED_EDGE('',*,*,#1293,.T.) ;
#1741=ORIENTED_EDGE('',*,*,#1294,.F.) ;
#1742=ORIENTED_EDGE('',*,*,#1295,.F.) ;
#1743=ORIENTED_EDGE('',*,*,#1293,.F.) ;
#1744=ORIENTED_EDGE('',*,*,#1288,.F.) ;
#1745=ORIENTED_EDGE('',*,*,#1294,.T.) ;
#1746=ORIENTED_EDGE('',*,*,#1295,.T.) ;
#1747=ORIENTED_EDGE('',*,*,#1296,.T.) ;
#1748=ORIENTED_EDGE('',*,*,#1292,.F.) ;
#1749=ORIENTED_EDGE('',*,*,#1290,.F.) ;
#1750=ORIENTED_EDGE('',*,*,#1296,.F.) ;
#2023=SPHERICAL_SURFACE('',#2360,6.5000000000005) ;
#2044=ADVANCED_FACE('',(#498),#463,.T.) ;
#2045=ADVANCED_FACE('',(#499,#87),#119,.F.) ;
#2046=ADVANCED_FACE('',(#500),#181,.T.) ;
#2047=ADVANCED_FACE('',(#501),#182,.F.) ;
#2048=ADVANCED_FACE('',(#502),#464,.T.) ;
#2049=ADVANCED_FACE('',(#503),#465,.F.) ;
#2050=ADVANCED_FACE('',(#504,#88),#120,.F.) ;
#2051=ADVANCED_FACE('',(#505),#183,.F.) ;
#2052=ADVANCED_FACE('',(#506),#184,.T.) ;
#2053=ADVANCED_FACE('',(#507,#89),#121,.F.) ;
#2054=ADVANCED_FACE('',(#508,#90),#122,.T.) ;
#2055=ADVANCED_FACE('',(#509,#91),#123,.F.) ;
#2056=ADVANCED_FACE('',(#510),#185,.F.) ;
#2057=ADVANCED_FACE('',(#511),#124,.F.) ;
#2058=ADVANCED_FACE('',(#512),#125,.F.) ;
#2059=ADVANCED_FACE('',(#513),#126,.T.) ;
#2060=ADVANCED_FACE('',(#514),#186,.F.) ;
#2061=ADVANCED_FACE('',(#515,#92),#127,.F.) ;
#2062=ADVANCED_FACE('',(#516,#93),#128,.F.) ;
#2063=ADVANCED_FACE('',(#517,#94),#129,.F.) ;
#2064=ADVANCED_FACE('',(#518,#95),#130,.F.) ;
#2065=ADVANCED_FACE('',(#519,#96),#131,.F.) ;
#2066=ADVANCED_FACE('',(#520),#187,.F.) ;
#2067=ADVANCED_FACE('',(#521),#132,.F.) ;
#2068=ADVANCED_FACE('',(#522),#133,.F.) ;
#2069=ADVANCED_FACE('',(#523),#134,.T.) ;
#2070=ADVANCED_FACE('',(#524),#188,.F.) ;
#2071=ADVANCED_FACE('',(#525),#189,.F.) ;
#2072=ADVANCED_FACE('',(#526),#135,.F.) ;
#2073=ADVANCED_FACE('',(#527),#136,.F.) ;
#2074=ADVANCED_FACE('',(#528),#137,.T.) ;
#2075=ADVANCED_FACE('',(#529),#190,.F.) ;
#2076=ADVANCED_FACE('',(#530),#191,.F.) ;
#2077=ADVANCED_FACE('',(#531),#138,.F.) ;
#2078=ADVANCED_FACE('',(#532),#139,.F.) ;
#2079=ADVANCED_FACE('',(#533),#140,.T.) ;
#2080=ADVANCED_FACE('',(#534),#192,.F.) ;
#2081=ADVANCED_FACE('',(#535),#193,.F.) ;
#2082=ADVANCED_FACE('',(#536),#141,.F.) ;
#2083=ADVANCED_FACE('',(#537),#142,.F.) ;
#2084=ADVANCED_FACE('',(#538),#143,.T.) ;
#2085=ADVANCED_FACE('',(#539),#194,.F.) ;
#2086=ADVANCED_FACE('',(#540),#195,.F.) ;
#2087=ADVANCED_FACE('',(#541),#144,.F.) ;
#2088=ADVANCED_FACE('',(#542),#145,.F.) ;
#2089=ADVANCED_FACE('',(#543),#146,.T.) ;
#2090=ADVANCED_FACE('',(#544),#196,.F.) ;
#2091=ADVANCED_FACE('',(#545,#97),#147,.T.) ;
#2092=ADVANCED_FACE('',(#546),#167,.T.) ;
#2093=ADVANCED_FACE('',(#547),#197,.T.) ;
#2094=ADVANCED_FACE('',(#548),#2023,.T.) ;
#2095=ADVANCED_FACE('',(#549),#168,.F.) ;
#2163=CLOSED_SHELL('',(#2044,#2045,#2046,#2047,#2048,#2049,#2050,#2051,
#2052,#2053,#2054,#2055,#2056,#2057,#2058,#2059,#2060,#2061,#2062,#2063,
#2064,#2065,#2066,#2067,#2068,#2069,#2070,#2071,#2072,#2073,#2074,#2075,
#2076,#2077,#2078,#2079,#2080,#2081,#2082,#2083,#2084,#2085,#2086,#2087,
#2088,#2089,#2090,#2091,#2092,#2093,#2094,#2095)) ;
#2268=AXIS2_PLACEMENT_3D('',#3369,#2646,#2647) ;
#2269=AXIS2_PLACEMENT_3D('',#3370,#2648,#2649) ;
#2270=AXIS2_PLACEMENT_3D('',#3372,#2650,#2651) ;
#2271=AXIS2_PLACEMENT_3D('',#3375,#2653,#2654) ;
#2272=AXIS2_PLACEMENT_3D('',#3376,#2655,#2656) ;
#2273=AXIS2_PLACEMENT_3D('',#3378,#2657,#2658) ;
#2274=AXIS2_PLACEMENT_3D('',#3379,#2659,#2660) ;
#2275=AXIS2_PLACEMENT_3D('',#3381,#2661,#2662) ;
#2276=AXIS2_PLACEMENT_3D('',#3383,#2664,#2665) ;
#2277=AXIS2_PLACEMENT_3D('',#3386,#2667,#2668) ;
#2278=AXIS2_PLACEMENT_3D('',#3387,#2669,#2670) ;
#2279=AXIS2_PLACEMENT_3D('',#3390,#2672,#2673) ;
#2280=AXIS2_PLACEMENT_3D('',#3391,#2674,#2675) ;
#2281=AXIS2_PLACEMENT_3D('',#3394,#2677,#2678) ;
#2282=AXIS2_PLACEMENT_3D('',#3395,#2679,#2680) ;
#2283=AXIS2_PLACEMENT_3D('',#3397,#2681,#2682) ;
#2284=AXIS2_PLACEMENT_3D('',#3398,#2683,#2684) ;
#2285=AXIS2_PLACEMENT_3D('',#3401,#2686,#2687) ;
#2286=AXIS2_PLACEMENT_3D('',#3402,#2688,#2689) ;
#2287=AXIS2_PLACEMENT_3D('',#3404,#2690,#2691) ;
#2288=AXIS2_PLACEMENT_3D('',#3406,#2693,#2694) ;
#2289=AXIS2_PLACEMENT_3D('',#3419,#2701,#2702) ;
#2290=AXIS2_PLACEMENT_3D('',#3433,#2709,#2710) ;
#2291=AXIS2_PLACEMENT_3D('',#3434,#2711,#2712) ;
#2292=AXIS2_PLACEMENT_3D('',#3439,#2715,#2716) ;
#2293=AXIS2_PLACEMENT_3D('',#3443,#2718,#2719) ;
#2294=AXIS2_PLACEMENT_3D('',#3445,#2721,#2722) ;
#2295=AXIS2_PLACEMENT_3D('',#3450,#2725,#2726) ;
#2296=AXIS2_PLACEMENT_3D('',#3451,#2727,#2728) ;
#2297=AXIS2_PLACEMENT_3D('',#3455,#2731,#2732) ;
#2298=AXIS2_PLACEMENT_3D('',#3459,#2735,#2736) ;
#2299=AXIS2_PLACEMENT_3D('',#3460,#2737,#2738) ;
#2300=AXIS2_PLACEMENT_3D('',#3461,#2739,#2740) ;
#2301=AXIS2_PLACEMENT_3D('',#3462,#2741,#2742) ;
#2302=AXIS2_PLACEMENT_3D('',#3468,#2745,#2746) ;
#2303=AXIS2_PLACEMENT_3D('',#3471,#2748,#2749) ;
#2304=AXIS2_PLACEMENT_3D('',#3472,#2750,#2751) ;
#2305=AXIS2_PLACEMENT_3D('',#3478,#2754,#2755) ;
#2306=AXIS2_PLACEMENT_3D('',#3481,#2757,#2758) ;
#2307=AXIS2_PLACEMENT_3D('',#3482,#2759,#2760) ;
#2308=AXIS2_PLACEMENT_3D('',#3488,#2763,#2764) ;
#2309=AXIS2_PLACEMENT_3D('',#3491,#2766,#2767) ;
#2310=AXIS2_PLACEMENT_3D('',#3492,#2768,#2769) ;
#2311=AXIS2_PLACEMENT_3D('',#3498,#2772,#2773) ;
#2312=AXIS2_PLACEMENT_3D('',#3501,#2775,#2776) ;
#2313=AXIS2_PLACEMENT_3D('',#3502,#2777,#2778) ;
#2314=AXIS2_PLACEMENT_3D('',#3507,#2780,#2781) ;
#2315=AXIS2_PLACEMENT_3D('',#3510,#2783,#2784) ;
#2316=AXIS2_PLACEMENT_3D('',#3511,#2785,#2786) ;
#2317=AXIS2_PLACEMENT_3D('',#3516,#2789,#2790) ;
#2318=AXIS2_PLACEMENT_3D('',#3517,#2791,#2792) ;
#2319=AXIS2_PLACEMENT_3D('',#3521,#2795,#2796) ;
#2320=AXIS2_PLACEMENT_3D('',#3525,#2799,#2800) ;
#2321=AXIS2_PLACEMENT_3D('',#3526,#2801,#2802) ;
#2322=AXIS2_PLACEMENT_3D('',#3527,#2803,#2804) ;
#2323=AXIS2_PLACEMENT_3D('',#3528,#2805,#2806) ;
#2324=AXIS2_PLACEMENT_3D('',#3533,#2809,#2810) ;
#2325=AXIS2_PLACEMENT_3D('',#3534,#2811,#2812) ;
#2326=AXIS2_PLACEMENT_3D('',#3538,#2815,#2816) ;
#2327=AXIS2_PLACEMENT_3D('',#3542,#2819,#2820) ;
#2328=AXIS2_PLACEMENT_3D('',#3543,#2821,#2822) ;
#2329=AXIS2_PLACEMENT_3D('',#3544,#2823,#2824) ;
#2330=AXIS2_PLACEMENT_3D('',#3545,#2825,#2826) ;
#2331=AXIS2_PLACEMENT_3D('',#3550,#2829,#2830) ;
#2332=AXIS2_PLACEMENT_3D('',#3551,#2831,#2832) ;
#2333=AXIS2_PLACEMENT_3D('',#3555,#2835,#2836) ;
#2334=AXIS2_PLACEMENT_3D('',#3559,#2839,#2840) ;
#2335=AXIS2_PLACEMENT_3D('',#3560,#2841,#2842) ;
#2336=AXIS2_PLACEMENT_3D('',#3561,#2843,#2844) ;
#2337=AXIS2_PLACEMENT_3D('',#3562,#2845,#2846) ;
#2338=AXIS2_PLACEMENT_3D('',#3567,#2849,#2850) ;
#2339=AXIS2_PLACEMENT_3D('',#3568,#2851,#2852) ;
#2340=AXIS2_PLACEMENT_3D('',#3572,#2855,#2856) ;
#2341=AXIS2_PLACEMENT_3D('',#3576,#2859,#2860) ;
#2342=AXIS2_PLACEMENT_3D('',#3577,#2861,#2862) ;
#2343=AXIS2_PLACEMENT_3D('',#3578,#2863,#2864) ;
#2344=AXIS2_PLACEMENT_3D('',#3579,#2865,#2866) ;
#2345=AXIS2_PLACEMENT_3D('',#3584,#2869,#2870) ;
#2346=AXIS2_PLACEMENT_3D('',#3585,#2871,#2872) ;
#2347=AXIS2_PLACEMENT_3D('',#3589,#2875,#2876) ;
#2348=AXIS2_PLACEMENT_3D('',#3593,#2879,#2880) ;
#2349=AXIS2_PLACEMENT_3D('',#3594,#2881,#2882) ;
#2350=AXIS2_PLACEMENT_3D('',#3595,#2883,#2884) ;
#2351=AXIS2_PLACEMENT_3D('',#3596,#2885,#2886) ;
#2352=AXIS2_PLACEMENT_3D('',#3598,#2887,#2888) ;
#2353=AXIS2_PLACEMENT_3D('',#3599,#2889,#2890) ;
#2354=AXIS2_PLACEMENT_3D('',#3601,#2891,#2892) ;
#2355=AXIS2_PLACEMENT_3D('',#3603,#2893,#2894) ;
#2356=AXIS2_PLACEMENT_3D('',#3604,#2895,#2896) ;
#2357=AXIS2_PLACEMENT_3D('',#3605,#2897,#2898) ;
#2358=AXIS2_PLACEMENT_3D('',#3608,#2899,#2900) ;
#2359=AXIS2_PLACEMENT_3D('',#3610,#2902,#2903) ;
#2360=AXIS2_PLACEMENT_3D('',#3611,#2904,#2905) ;
#2361=AXIS2_PLACEMENT_3D('',#3613,#2906,#2907) ;
#2362=AXIS2_PLACEMENT_3D('',#3615,#2908,#2909) ;
#2363=AXIS2_PLACEMENT_3D('',#3616,#2910,#2911) ;
#2364=AXIS2_PLACEMENT_3D('',#3617,#2912,#2913) ;
#2365=AXIS2_PLACEMENT_3D('',#3618,#2914,#2915) ;
#2646=DIRECTION('axis',(0.,0.,1.)) ;
#2647=DIRECTION('refdir',(1.,0.,0.)) ;
#2648=DIRECTION('center_axis',(-0.855521240266964,0.510121382366096,-0.0886542875724541)) ;
#2649=DIRECTION('ref_axis',(0.442722751678459,0.631934937682125,-0.636124830267568)) ;
#2650=DIRECTION('center_axis',(-0.855521240266964,0.510121382366096,-0.0886542875724541)) ;
#2651=DIRECTION('ref_axis',(0.517240562193751,0.834304337432909,-0.190783839363105)) ;
#2652=DIRECTION('',(0.811169769918609,0.292211018391187,-0.506573119204895)) ;
#2653=DIRECTION('center_axis',(-0.855521240266964,0.510121382366096,-0.0886542875724541)) ;
#2654=DIRECTION('ref_axis',(0.517240562193751,0.834304337432909,-0.190783839363105)) ;
#2655=DIRECTION('center_axis',(-0.855521240266964,0.510121382366096,-0.0886542875724541)) ;
#2656=DIRECTION('ref_axis',(0.0233582592152952,0.209075220419679,0.977620552122803)) ;
#2657=DIRECTION('center_axis',(-0.855521240266964,0.510121382366096,-0.0886542875724541)) ;
#2658=DIRECTION('ref_axis',(0.517240562193751,0.834304337432909,-0.190783839363105)) ;
#2659=DIRECTION('center_axis',(-0.855521240266964,0.510121382366096,-0.0886542875724541)) ;
#2660=DIRECTION('ref_axis',(0.442722751678459,0.631934937682125,-0.636124830267568)) ;
#2661=DIRECTION('center_axis',(-0.855521240266964,0.510121382366096,-0.0886542875724541)) ;
#2662=DIRECTION('ref_axis',(0.517240562193751,0.834304337432909,-0.190783839363105)) ;
#2663=DIRECTION('',(0.855521240266964,-0.510121382366096,0.0886542875724541)) ;
#2664=DIRECTION('center_axis',(-0.855521240266964,0.510121382366096,-0.0886542875724541)) ;
#2665=DIRECTION('ref_axis',(0.442722751678459,0.631934937682125,-0.636124830267568)) ;
#2666=DIRECTION('',(-0.855521240266964,0.510121382366096,-0.0886542875724541)) ;
#2667=DIRECTION('center_axis',(-0.855521240266964,0.510121382366096,-0.0886542875724541)) ;
#2668=DIRECTION('ref_axis',(0.517240562193751,0.834304337432909,-0.190783839363105)) ;
#2669=DIRECTION('center_axis',(0.855521240266964,-0.510121382366096,0.0886542875724541)) ;
#2670=DIRECTION('ref_axis',(0.442722751678459,0.631934937682125,-0.636124830267568)) ;
#2671=DIRECTION('',(-0.0443514703433129,0.802332400754277,-0.595227406776826)) ;
#2672=DIRECTION('center_axis',(0.855521240266964,-0.510121382366096,0.0886542875724541)) ;
#2673=DIRECTION('ref_axis',(-0.517240562193751,-0.834304337432909,0.190783839363105)) ;
#2674=DIRECTION('center_axis',(-0.855521240266964,0.510121382366096,-0.0886542875724541)) ;
#2675=DIRECTION('ref_axis',(0.442722751678459,0.631934937682125,-0.636124830267568)) ;
#2676=DIRECTION('',(-0.917997130339433,-0.0861351910040448,0.387120133239365)) ;
#2677=DIRECTION('center_axis',(-0.855521240266964,0.510121382366096,-0.0886542875724541)) ;
#2678=DIRECTION('ref_axis',(0.517240562193751,0.834304337432909,-0.190783839363105)) ;
#2679=DIRECTION('center_axis',(-0.855521240266964,0.510121382366096,-0.0886542875724541)) ;
#2680=DIRECTION('ref_axis',(0.0233582592152952,0.209075220419679,0.977620552122803)) ;
#2681=DIRECTION('center_axis',(-0.855521240266964,0.510121382366096,-0.0886542875724541)) ;
#2682=DIRECTION('ref_axis',(0.517240562193751,0.834304337432909,-0.190783839363105)) ;
#2683=DIRECTION('center_axis',(-0.855521240266964,0.510121382366096,-0.0886542875724541)) ;
#2684=DIRECTION('ref_axis',(0.442722751678459,0.631934937682125,-0.636124830267568)) ;
#2685=DIRECTION('',(-0.855521240266964,0.510121382366096,-0.0886542875724541)) ;
#2686=DIRECTION('center_axis',(-0.855521240266964,0.510121382366096,-0.0886542875724541)) ;
#2687=DIRECTION('ref_axis',(0.517240562193751,0.834304337432909,-0.190783839363105)) ;
#2688=DIRECTION('center_axis',(-0.855521240266964,0.510121382366096,-0.0886542875724541)) ;
#2689=DIRECTION('ref_axis',(0.442722751678459,0.631934937682125,-0.636124830267568)) ;
#2690=DIRECTION('center_axis',(-0.855521240266964,0.510121382366096,-0.0886542875724541)) ;
#2691=DIRECTION('ref_axis',(0.517240562193751,0.834304337432909,-0.190783839363105)) ;
#2692=DIRECTION('',(0.855521240266964,-0.510121382366096,0.0886542875724541)) ;
#2693=DIRECTION('center_axis',(-0.855521240266964,0.510121382366096,-0.0886542875724541)) ;
#2694=DIRECTION('ref_axis',(0.0233582592152952,0.209075220419679,0.977620552122803)) ;
#2695=DIRECTION('',(-0.0233582592152952,-0.209075220419679,-0.977620552122803)) ;
#2696=DIRECTION('',(0.436264337119824,0.617991140494473,-0.654033927581544)) ;
#2697=DIRECTION('',(0.459622596335128,0.827066360914232,0.32358662454163)) ;
#2698=DIRECTION('',(0.0233582592152952,0.209075220419679,0.977620552122803)) ;
#2699=DIRECTION('',(-0.436264337119824,-0.617991140494473,0.654033927581544)) ;
#2700=DIRECTION('',(-0.459622596335128,-0.827066360914232,-0.32358662454163)) ;
#2701=DIRECTION('center_axis',(-0.855521240266964,0.510121382366096,-0.0886542875724541)) ;
#2702=DIRECTION('ref_axis',(0.0233582592152952,0.209075220419679,0.977620552122803)) ;
#2703=DIRECTION('',(-0.436264337119824,-0.617991140494473,0.654033927581544)) ;
#2704=DIRECTION('',(0.0233582592152952,0.209075220419679,0.977620552122803)) ;
#2705=DIRECTION('',(0.459622596335128,0.827066360914232,0.32358662454163)) ;
#2706=DIRECTION('',(0.436264337119824,0.617991140494473,-0.654033927581544)) ;
#2707=DIRECTION('',(-0.0233582592152952,-0.209075220419679,-0.977620552122803)) ;
#2708=DIRECTION('',(-0.459622596335128,-0.827066360914232,-0.32358662454163)) ;
#2709=DIRECTION('center_axis',(-0.855521240266964,0.510121382366096,-0.0886542875724541)) ;
#2710=DIRECTION('ref_axis',(0.517240562193751,0.834304337432909,-0.190783839363105)) ;
#2711=DIRECTION('center_axis',(-0.51724056219375,-0.83430433743291,0.190783839363105)) ;
#2712=DIRECTION('ref_axis',(0.0233582592152955,0.209075220419679,0.977620552122803)) ;
#2713=DIRECTION('',(-0.855521240266964,0.510121382366096,-0.0886542875724541)) ;
#2714=DIRECTION('',(-0.855521240266964,0.510121382366096,-0.0886542875724541)) ;
#2715=DIRECTION('center_axis',(-0.51724056219375,-0.83430433743291,0.190783839363105)) ;
#2716=DIRECTION('ref_axis',(0.0233582592152955,0.209075220419679,0.977620552122803)) ;
#2717=DIRECTION('',(-0.023358259215295,-0.209075220419679,-0.977620552122803)) ;
#2718=DIRECTION('center_axis',(-0.51724056219375,-0.83430433743291,0.190783839363105)) ;
#2719=DIRECTION('ref_axis',(0.0233582592152955,0.209075220419679,0.977620552122803)) ;
#2720=DIRECTION('',(0.023358259215295,0.209075220419679,0.977620552122803)) ;
#2721=DIRECTION('center_axis',(0.51724056219375,0.83430433743291,-0.190783839363105)) ;
#2722=DIRECTION('ref_axis',(0.855521240266964,-0.510121382366095,0.088654287572454)) ;
#2723=DIRECTION('',(0.51724056219375,0.83430433743291,-0.190783839363105)) ;
#2724=DIRECTION('',(0.51724056219375,0.83430433743291,-0.190783839363105)) ;
#2725=DIRECTION('center_axis',(0.51724056219375,0.83430433743291,-0.190783839363105)) ;
#2726=DIRECTION('ref_axis',(-0.0233582592152955,-0.209075220419679,-0.977620552122803)) ;
#2727=DIRECTION('center_axis',(0.855521240266964,-0.510121382366096,0.0886542875724541)) ;
#2728=DIRECTION('ref_axis',(0.0233582592152952,0.209075220419679,0.977620552122803)) ;
#2729=DIRECTION('',(-0.51724056219375,-0.83430433743291,0.190783839363105)) ;
#2730=DIRECTION('',(0.0233582592152952,0.209075220419679,0.977620552122803)) ;
#2731=DIRECTION('center_axis',(-0.855521240266964,0.510121382366096,-0.0886542875724541)) ;
#2732=DIRECTION('ref_axis',(-0.0233582592152952,-0.209075220419679,-0.977620552122803)) ;
#2733=DIRECTION('',(-0.51724056219375,-0.83430433743291,0.190783839363105)) ;
#2734=DIRECTION('',(-0.0233582592152952,-0.209075220419679,-0.977620552122803)) ;
#2735=DIRECTION('center_axis',(0.51724056219375,0.83430433743291,-0.190783839363105)) ;
#2736=DIRECTION('ref_axis',(0.0233582592152955,0.209075220419679,0.977620552122803)) ;
#2737=DIRECTION('center_axis',(0.51724056219375,0.83430433743291,-0.190783839363105)) ;
#2738=DIRECTION('ref_axis',(-0.0233582592152955,-0.209075220419679,-0.977620552122803)) ;
#2739=DIRECTION('center_axis',(0.51724056219375,0.83430433743291,-0.190783839363105)) ;
#2740=DIRECTION('ref_axis',(-0.855521240266964,0.510121382366095,-0.0886542875724542)) ;
#2741=DIRECTION('center_axis',(-0.238391435228348,-0.236087716531363,0.942036153081598)) ;
#2742=DIRECTION('ref_axis',(0.459622596335128,0.827066360914232,0.323586624541629)) ;
#2743=DIRECTION('',(-0.855521240266964,0.510121382366096,-0.0886542875724541)) ;
#2744=DIRECTION('',(-0.459622596335128,-0.827066360914232,-0.32358662454163)) ;
#2745=DIRECTION('center_axis',(-0.238391435228348,-0.236087716531363,0.942036153081598)) ;
#2746=DIRECTION('ref_axis',(-0.855521240266964,0.510121382366096,-0.0886542875724536)) ;
#2747=DIRECTION('',(0.459622596335128,0.827066360914232,0.32358662454163)) ;
#2748=DIRECTION('center_axis',(-0.238391435228348,-0.236087716531363,0.942036153081598)) ;
#2749=DIRECTION('ref_axis',(-0.855521240266964,0.510121382366096,-0.0886542875724536)) ;
#2750=DIRECTION('center_axis',(-0.278849126965598,-0.598216620901864,-0.75125231371842)) ;
#2751=DIRECTION('ref_axis',(-0.436264337119824,-0.617991140494473,0.654033927581545)) ;
#2752=DIRECTION('',(-0.855521240266964,0.510121382366096,-0.0886542875724541)) ;
#2753=DIRECTION('',(0.436264337119824,0.617991140494473,-0.654033927581544)) ;
#2754=DIRECTION('center_axis',(-0.278849126965598,-0.598216620901864,-0.75125231371842)) ;
#2755=DIRECTION('ref_axis',(0.855521240266964,-0.510121382366095,0.0886542875724546)) ;
#2756=DIRECTION('',(-0.436264337119824,-0.617991140494473,0.654033927581544)) ;
#2757=DIRECTION('center_axis',(-0.278849126965598,-0.598216620901864,-0.75125231371842)) ;
#2758=DIRECTION('ref_axis',(0.855521240266964,-0.510121382366095,0.0886542875724546)) ;
#2759=DIRECTION('center_axis',(0.278849126965598,0.598216620901864,0.75125231371842)) ;
#2760=DIRECTION('ref_axis',(0.436264337119824,0.617991140494473,-0.654033927581545)) ;
#2761=DIRECTION('',(-0.855521240266964,0.510121382366096,-0.0886542875724541)) ;
#2762=DIRECTION('',(-0.436264337119824,-0.617991140494473,0.654033927581544)) ;
#2763=DIRECTION('center_axis',(0.278849126965598,0.598216620901864,0.75125231371842)) ;
#2764=DIRECTION('ref_axis',(-0.855521240266964,0.510121382366095,-0.0886542875724546)) ;
#2765=DIRECTION('',(0.436264337119824,0.617991140494473,-0.654033927581544)) ;
#2766=DIRECTION('center_axis',(0.278849126965598,0.598216620901864,0.75125231371842)) ;
#2767=DIRECTION('ref_axis',(-0.855521240266964,0.510121382366095,-0.0886542875724546)) ;
#2768=DIRECTION('center_axis',(0.238391435228348,0.236087716531363,-0.942036153081598)) ;
#2769=DIRECTION('ref_axis',(-0.459622596335128,-0.827066360914232,-0.323586624541629)) ;
#2770=DIRECTION('',(-0.855521240266964,0.510121382366096,-0.0886542875724541)) ;
#2771=DIRECTION('',(0.459622596335128,0.827066360914232,0.32358662454163)) ;
#2772=DIRECTION('center_axis',(0.238391435228348,0.236087716531363,-0.942036153081598)) ;
#2773=DIRECTION('ref_axis',(0.855521240266964,-0.510121382366096,0.0886542875724536)) ;
#2774=DIRECTION('',(-0.459622596335128,-0.827066360914232,-0.32358662454163)) ;
#2775=DIRECTION('center_axis',(0.238391435228348,0.236087716531363,-0.942036153081598)) ;
#2776=DIRECTION('ref_axis',(0.855521240266964,-0.510121382366096,0.0886542875724536)) ;
#2777=DIRECTION('center_axis',(0.51724056219375,0.83430433743291,-0.190783839363105)) ;
#2778=DIRECTION('ref_axis',(-0.0233582592152955,-0.209075220419679,-0.977620552122803)) ;
#2779=DIRECTION('',(0.0233582592152952,0.209075220419679,0.977620552122803)) ;
#2780=DIRECTION('center_axis',(0.51724056219375,0.83430433743291,-0.190783839363105)) ;
#2781=DIRECTION('ref_axis',(-0.0233582592152955,-0.209075220419679,-0.977620552122803)) ;
#2782=DIRECTION('',(-0.0233582592152952,-0.209075220419679,-0.977620552122803)) ;
#2783=DIRECTION('center_axis',(0.51724056219375,0.83430433743291,-0.190783839363105)) ;
#2784=DIRECTION('ref_axis',(-0.0233582592152955,-0.209075220419679,-0.977620552122803)) ;
#2785=DIRECTION('center_axis',(-0.51724056219375,-0.83430433743291,0.190783839363105)) ;
#2786=DIRECTION('ref_axis',(0.855521240266964,-0.510121382366095,0.088654287572454)) ;
#2787=DIRECTION('',(-0.51724056219375,-0.83430433743291,0.190783839363105)) ;
#2788=DIRECTION('',(-0.51724056219375,-0.83430433743291,0.190783839363105)) ;
#2789=DIRECTION('center_axis',(-0.51724056219375,-0.83430433743291,0.190783839363105)) ;
#2790=DIRECTION('ref_axis',(0.0233582592152956,0.209075220419679,0.977620552122803)) ;
#2791=DIRECTION('center_axis',(0.855521240266964,-0.510121382366096,0.0886542875724541)) ;
#2792=DIRECTION('ref_axis',(0.0233582592152952,0.209075220419679,0.977620552122803)) ;
#2793=DIRECTION('',(0.51724056219375,0.83430433743291,-0.190783839363105)) ;
#2794=DIRECTION('',(-0.0233582592152952,-0.209075220419679,-0.977620552122803)) ;
#2795=DIRECTION('center_axis',(-0.855521240266964,0.510121382366096,-0.0886542875724541)) ;
#2796=DIRECTION('ref_axis',(-0.0233582592152952,-0.209075220419679,-0.977620552122803)) ;
#2797=DIRECTION('',(0.51724056219375,0.83430433743291,-0.190783839363105)) ;
#2798=DIRECTION('',(0.0233582592152952,0.209075220419679,0.977620552122803)) ;
#2799=DIRECTION('center_axis',(-0.51724056219375,-0.83430433743291,0.190783839363105)) ;
#2800=DIRECTION('ref_axis',(-0.0233582592152955,-0.209075220419679,-0.977620552122803)) ;
#2801=DIRECTION('center_axis',(-0.51724056219375,-0.83430433743291,0.190783839363105)) ;
#2802=DIRECTION('ref_axis',(0.0233582592152956,0.209075220419679,0.977620552122803)) ;
#2803=DIRECTION('center_axis',(-0.51724056219375,-0.83430433743291,0.190783839363105)) ;
#2804=DIRECTION('ref_axis',(-0.855521240266964,0.510121382366095,-0.0886542875724539)) ;
#2805=DIRECTION('center_axis',(0.278849126965598,0.598216620901864,0.75125231371842)) ;
#2806=DIRECTION('ref_axis',(0.855521240266964,-0.510121382366095,0.0886542875724547)) ;
#2807=DIRECTION('',(0.278849126965598,0.598216620901864,0.75125231371842)) ;
#2808=DIRECTION('',(0.278849126965598,0.598216620901864,0.75125231371842)) ;
#2809=DIRECTION('center_axis',(0.278849126965598,0.598216620901864,0.75125231371842)) ;
#2810=DIRECTION('ref_axis',(-0.855521240266964,0.510121382366095,-0.0886542875724546)) ;
#2811=DIRECTION('center_axis',(0.855521240266964,-0.510121382366096,0.0886542875724541)) ;
#2812=DIRECTION('ref_axis',(0.0233582592152952,0.209075220419679,0.977620552122803)) ;
#2813=DIRECTION('',(-0.278849126965598,-0.598216620901864,-0.75125231371842)) ;
#2814=DIRECTION('',(-0.436264337119824,-0.617991140494473,0.654033927581544)) ;
#2815=DIRECTION('center_axis',(-0.855521240266964,0.510121382366096,-0.0886542875724541)) ;
#2816=DIRECTION('ref_axis',(-0.0233582592152952,-0.209075220419679,-0.977620552122803)) ;
#2817=DIRECTION('',(-0.278849126965598,-0.598216620901864,-0.75125231371842)) ;
#2818=DIRECTION('',(0.436264337119824,0.617991140494473,-0.654033927581544)) ;
#2819=DIRECTION('center_axis',(0.278849126965598,0.598216620901864,0.75125231371842)) ;
#2820=DIRECTION('ref_axis',(-0.436264337119824,-0.617991140494473,0.654033927581545)) ;
#2821=DIRECTION('center_axis',(0.278849126965598,0.598216620901864,0.75125231371842)) ;
#2822=DIRECTION('ref_axis',(-0.855521240266964,0.510121382366095,-0.0886542875724546)) ;
#2823=DIRECTION('center_axis',(0.278849126965598,0.598216620901864,0.75125231371842)) ;
#2824=DIRECTION('ref_axis',(-0.855521240266964,0.510121382366095,-0.0886542875724547)) ;
#2825=DIRECTION('center_axis',(-0.278849126965598,-0.598216620901864,-0.75125231371842)) ;
#2826=DIRECTION('ref_axis',(0.855521240266964,-0.510121382366095,0.0886542875724546)) ;
#2827=DIRECTION('',(-0.278849126965598,-0.598216620901864,-0.75125231371842)) ;
#2828=DIRECTION('',(-0.278849126965598,-0.598216620901864,-0.75125231371842)) ;
#2829=DIRECTION('center_axis',(-0.278849126965598,-0.598216620901864,-0.75125231371842)) ;
#2830=DIRECTION('ref_axis',(0.855521240266964,-0.510121382366095,0.0886542875724546)) ;
#2831=DIRECTION('center_axis',(0.855521240266964,-0.510121382366096,0.0886542875724541)) ;
#2832=DIRECTION('ref_axis',(0.0233582592152952,0.209075220419679,0.977620552122803)) ;
#2833=DIRECTION('',(0.278849126965598,0.598216620901864,0.75125231371842)) ;
#2834=DIRECTION('',(0.436264337119824,0.617991140494473,-0.654033927581544)) ;
#2835=DIRECTION('center_axis',(-0.855521240266964,0.510121382366096,-0.0886542875724541)) ;
#2836=DIRECTION('ref_axis',(-0.0233582592152952,-0.209075220419679,-0.977620552122803)) ;
#2837=DIRECTION('',(0.278849126965598,0.598216620901864,0.75125231371842)) ;
#2838=DIRECTION('',(-0.436264337119824,-0.617991140494473,0.654033927581544)) ;
#2839=DIRECTION('center_axis',(-0.278849126965598,-0.598216620901864,-0.75125231371842)) ;
#2840=DIRECTION('ref_axis',(0.436264337119824,0.617991140494473,-0.654033927581545)) ;
#2841=DIRECTION('center_axis',(-0.278849126965598,-0.598216620901864,-0.75125231371842)) ;
#2842=DIRECTION('ref_axis',(0.855521240266964,-0.510121382366095,0.0886542875724546)) ;
#2843=DIRECTION('center_axis',(-0.278849126965598,-0.598216620901864,-0.75125231371842)) ;
#2844=DIRECTION('ref_axis',(-0.855521240266964,0.510121382366095,-0.0886542875724546)) ;
#2845=DIRECTION('center_axis',(0.238391435228348,0.236087716531363,-0.942036153081598)) ;
#2846=DIRECTION('ref_axis',(0.855521240266964,-0.510121382366096,0.0886542875724536)) ;
#2847=DIRECTION('',(0.238391435228348,0.236087716531363,-0.942036153081598)) ;
#2848=DIRECTION('',(0.238391435228348,0.236087716531363,-0.942036153081598)) ;
#2849=DIRECTION('center_axis',(0.238391435228348,0.236087716531363,-0.942036153081598)) ;
#2850=DIRECTION('ref_axis',(0.855521240266964,-0.510121382366096,0.0886542875724536)) ;
#2851=DIRECTION('center_axis',(0.855521240266964,-0.510121382366096,0.0886542875724541)) ;
#2852=DIRECTION('ref_axis',(0.0233582592152952,0.209075220419679,0.977620552122803)) ;
#2853=DIRECTION('',(-0.238391435228348,-0.236087716531363,0.942036153081598)) ;
#2854=DIRECTION('',(0.459622596335128,0.827066360914232,0.32358662454163)) ;
#2855=DIRECTION('center_axis',(-0.855521240266964,0.510121382366096,-0.0886542875724541)) ;
#2856=DIRECTION('ref_axis',(-0.0233582592152952,-0.209075220419679,-0.977620552122803)) ;
#2857=DIRECTION('',(-0.238391435228348,-0.236087716531363,0.942036153081598)) ;
#2858=DIRECTION('',(-0.459622596335128,-0.827066360914232,-0.32358662454163)) ;
#2859=DIRECTION('center_axis',(0.238391435228348,0.236087716531363,-0.942036153081598)) ;
#2860=DIRECTION('ref_axis',(0.459622596335128,0.827066360914232,0.323586624541629)) ;
#2861=DIRECTION('center_axis',(0.238391435228348,0.236087716531363,-0.942036153081598)) ;
#2862=DIRECTION('ref_axis',(0.855521240266964,-0.510121382366096,0.0886542875724536)) ;
#2863=DIRECTION('center_axis',(0.238391435228348,0.236087716531363,-0.942036153081598)) ;
#2864=DIRECTION('ref_axis',(-0.855521240266964,0.510121382366096,-0.0886542875724537)) ;
#2865=DIRECTION('center_axis',(-0.238391435228348,-0.236087716531363,0.942036153081598)) ;
#2866=DIRECTION('ref_axis',(0.855521240266964,-0.510121382366096,0.0886542875724536)) ;
#2867=DIRECTION('',(-0.238391435228348,-0.236087716531363,0.942036153081598)) ;
#2868=DIRECTION('',(-0.238391435228348,-0.236087716531363,0.942036153081598)) ;
#2869=DIRECTION('center_axis',(-0.238391435228348,-0.236087716531363,0.942036153081598)) ;
#2870=DIRECTION('ref_axis',(-0.855521240266964,0.510121382366096,-0.0886542875724536)) ;
#2871=DIRECTION('center_axis',(0.855521240266964,-0.510121382366096,0.0886542875724541)) ;
#2872=DIRECTION('ref_axis',(0.0233582592152952,0.209075220419679,0.977620552122803)) ;
#2873=DIRECTION('',(0.238391435228348,0.236087716531363,-0.942036153081598)) ;
#2874=DIRECTION('',(-0.459622596335128,-0.827066360914232,-0.32358662454163)) ;
#2875=DIRECTION('center_axis',(-0.855521240266964,0.510121382366096,-0.0886542875724541)) ;
#2876=DIRECTION('ref_axis',(-0.0233582592152952,-0.209075220419679,-0.977620552122803)) ;
#2877=DIRECTION('',(0.238391435228348,0.236087716531363,-0.942036153081598)) ;
#2878=DIRECTION('',(0.459622596335128,0.827066360914232,0.32358662454163)) ;
#2879=DIRECTION('center_axis',(-0.238391435228348,-0.236087716531363,0.942036153081598)) ;
#2880=DIRECTION('ref_axis',(-0.459622596335128,-0.827066360914232,-0.323586624541629)) ;
#2881=DIRECTION('center_axis',(-0.238391435228348,-0.236087716531363,0.942036153081598)) ;
#2882=DIRECTION('ref_axis',(-0.855521240266964,0.510121382366096,-0.0886542875724536)) ;
#2883=DIRECTION('center_axis',(-0.238391435228348,-0.236087716531363,0.942036153081598)) ;
#2884=DIRECTION('ref_axis',(-0.855521240266964,0.510121382366096,-0.0886542875724536)) ;
#2885=DIRECTION('center_axis',(-0.855521240266964,0.510121382366096,-0.0886542875724541)) ;
#2886=DIRECTION('ref_axis',(0.0233582592152952,0.209075220419679,0.977620552122803)) ;
#2887=DIRECTION('center_axis',(-0.855521240266964,0.510121382366096,-0.0886542875724541)) ;
#2888=DIRECTION('ref_axis',(0.517240562193751,0.834304337432909,-0.190783839363105)) ;
#2889=DIRECTION('center_axis',(-0.855521240266964,0.510121382366096,-0.0886542875724543)) ;
#2890=DIRECTION('ref_axis',(-0.509251476733416,-0.798095832523249,0.322034121722927)) ;
#2891=DIRECTION('center_axis',(-0.093521873895457,-0.320654358089701,-0.942568003775411)) ;
#2892=DIRECTION('ref_axis',(0.509251476733411,0.798095832523253,-0.322034121722926)) ;
#2893=DIRECTION('center_axis',(-0.855521240266964,0.510121382366096,-0.0886542875724543)) ;
#2894=DIRECTION('ref_axis',(0.517240562193751,0.834304337432909,-0.190783839363105)) ;
#2895=DIRECTION('center_axis',(-0.855521240266964,0.510121382366096,-0.0886542875724543)) ;
#2896=DIRECTION('ref_axis',(0.517240562193751,0.834304337432909,-0.190783839363105)) ;
#2897=DIRECTION('center_axis',(-0.855521240266964,0.510121382366096,-0.0886542875724541)) ;
#2898=DIRECTION('ref_axis',(0.442722751678459,0.631934937682125,-0.636124830267568)) ;
#2899=DIRECTION('center_axis',(-0.855521240266964,0.510121382366096,-0.0886542875724541)) ;
#2900=DIRECTION('ref_axis',(0.517240562193751,0.834304337432909,-0.190783839363105)) ;
#2901=DIRECTION('',(0.855521240266964,-0.510121382366096,0.0886542875724541)) ;
#2902=DIRECTION('center_axis',(-0.855521240266964,0.510121382366096,-0.0886542875724541)) ;
#2903=DIRECTION('ref_axis',(0.517240562193751,0.834304337432909,-0.190783839363105)) ;
#2904=DIRECTION('center_axis',(-0.855521240266964,0.510121382366095,-0.088654287572454)) ;
#2905=DIRECTION('ref_axis',(0.442722751678459,0.631934937682125,-0.636124830267568)) ;
#2906=DIRECTION('center_axis',(0.268477136081137,0.583467573897292,0.766476103744976)) ;
#2907=DIRECTION('ref_axis',(-0.442722751678459,-0.631934937682125,0.636124830267568)) ;
#2908=DIRECTION('center_axis',(-0.855521240266964,0.510121382366096,-0.0886542875724541)) ;
#2909=DIRECTION('ref_axis',(0.51724056219375,0.834304337432909,-0.190783839363105)) ;
#2910=DIRECTION('center_axis',(-0.855521240266964,0.510121382366096,-0.0886542875724541)) ;
#2911=DIRECTION('ref_axis',(0.51724056219375,0.834304337432909,-0.190783839363105)) ;
#2912=DIRECTION('center_axis',(-0.855521240266964,0.510121382366096,-0.0886542875724541)) ;
#2913=DIRECTION('ref_axis',(-0.515977131070524,-0.85419973905181,0.06411244821445)) ;
#2914=DIRECTION('center_axis',(-0.0430233386001843,0.100593146171714,0.99399698756031)) ;
#2915=DIRECTION('ref_axis',(0.515977131070522,0.854199739051811,-0.0641124482144504)) ;
#3369=CARTESIAN_POINT('',(0.,0.,0.)) ;
#3370=CARTESIAN_POINT('Origin',(-415.730955726499,145.572172760385,-57.8683245658292)) ;
#3371=CARTESIAN_POINT('',(-418.171335668733,142.669556598323,-54.8039516305242)) ;
#3372=CARTESIAN_POINT('Origin',(-416.01793220457,145.743288135211,-57.8980628049471)) ;
#3373=CARTESIAN_POINT('',(-417.627137271938,142.865595422292,-55.143801917793)) ;
#3374=CARTESIAN_POINT('',(-417.627137271938,142.865595422292,-55.143801917793)) ;
#3375=CARTESIAN_POINT('Origin',(-415.730955726499,145.572172760385,-57.8683245658292)) ;
#3376=CARTESIAN_POINT('Origin',(-414.179234039917,148.075085772684,-58.4406760839186)) ;
#3377=CARTESIAN_POINT('',(-417.059123981534,143.676367947338,-55.9599500750264)) ;
#3378=CARTESIAN_POINT('Origin',(-415.730955726499,145.572172760385,-57.8683245658292)) ;
#3379=CARTESIAN_POINT('Origin',(-426.211090919796,151.821159694385,-58.9543395885945)) ;
#3380=CARTESIAN_POINT('',(-424.869313254862,146.663357598784,-55.4980365966556)) ;
#3381=CARTESIAN_POINT('Origin',(-422.715909790697,149.73708913567,-58.5921477710773)) ;
#3382=CARTESIAN_POINT('',(-428.36449438396,148.747428157499,-55.8602284141728)) ;
#3383=CARTESIAN_POINT('Origin',(-426.211090919796,151.821159694385,-58.9543395885945)) ;
#3384=CARTESIAN_POINT('',(-432.372954182314,152.807540691692,-57.5468618225734)) ;
#3385=CARTESIAN_POINT('',(-427.539259174831,149.925354881338,-57.0459650977917)) ;
#3386=CARTESIAN_POINT('Origin',(-431.044785927279,154.703345504738,-59.4552363133763)) ;
#3387=CARTESIAN_POINT('Origin',(-423.002886268769,149.908204510497,-58.6218860101951)) ;
#3388=CARTESIAN_POINT('',(-424.899067814208,147.201627172404,-55.8973633621589)) ;
#3389=CARTESIAN_POINT('',(-424.899067814208,147.201627172404,-55.8973633621589)) ;
#3390=CARTESIAN_POINT('Origin',(-423.002886268769,149.908204510497,-58.6218860101951)) ;
#3391=CARTESIAN_POINT('Origin',(-431.044785927279,154.703345504738,-59.4552363133763)) ;
#3392=CARTESIAN_POINT('',(-433.801022573454,152.673545780845,-56.9446442256091)) ;
#3393=CARTESIAN_POINT('',(-432.372954182314,152.807540691691,-57.5468618225734)) ;
#3394=CARTESIAN_POINT('Origin',(-431.985859291572,155.264479025341,-59.552756029706)) ;
#3395=CARTESIAN_POINT('Origin',(-420.787544940893,153.481529987722,-59.4390131941874)) ;
#3396=CARTESIAN_POINT('',(-425.15628973293,146.834472973614,-55.5277748357752)) ;
#3397=CARTESIAN_POINT('Origin',(-423.002886268769,149.908204510497,-58.6218860101951)) ;
#3398=CARTESIAN_POINT('Origin',(-426.211090919796,151.821159694385,-58.9543395885945)) ;
#3399=CARTESIAN_POINT('',(-438.506389394923,155.479213383858,-57.4322428072573)) ;
#3400=CARTESIAN_POINT('',(-428.026254201678,149.230226449888,-56.3462277844973)) ;
#3401=CARTESIAN_POINT('Origin',(-436.691226113041,158.070146628355,-60.0403546113545)) ;
#3402=CARTESIAN_POINT('Origin',(-426.211090919796,151.821159694385,-58.9543395885945)) ;
#3403=CARTESIAN_POINT('',(-426.011810973197,147.344594355981,-55.6164291233476)) ;
#3404=CARTESIAN_POINT('Origin',(-423.858407509036,150.418325892863,-58.7105402977676)) ;
#3405=CARTESIAN_POINT('',(-428.36449438396,148.747428157499,-55.8602284141728)) ;
#3406=CARTESIAN_POINT('Origin',(-421.342549414525,154.476382190137,-59.6385128924298)) ;
#3407=CARTESIAN_POINT('',(-427.233563764187,145.637241385156,-53.650610998181)) ;
#3408=CARTESIAN_POINT('',(-427.414274787281,144.019732278968,-61.2139661498883)) ;
#3409=CARTESIAN_POINT('',(-427.323919275734,144.828486832062,-57.4322885740347)) ;
#3410=CARTESIAN_POINT('',(-424.039118532129,148.800816786675,-66.2738954494749)) ;
#3411=CARTESIAN_POINT('',(-425.726696659705,146.41027453282,-63.7439307996865)) ;
#3412=CARTESIAN_POINT('',(-420.483251253884,155.19941040057,-63.7704695973542)) ;
#3413=CARTESIAN_POINT('',(-422.261184893006,152.000113593621,-65.0221825234194)) ;
#3414=CARTESIAN_POINT('',(-420.302540230791,156.816919506758,-56.2071144456468)) ;
#3415=CARTESIAN_POINT('',(-420.392895742337,156.008164953664,-59.9887920215005)) ;
#3416=CARTESIAN_POINT('',(-423.677696485943,152.035834999051,-51.1471851460603)) ;
#3417=CARTESIAN_POINT('',(-421.990118358366,154.426377252906,-53.6771497958487)) ;
#3418=CARTESIAN_POINT('',(-425.455630125065,148.836538192105,-52.3988980721158)) ;
#3419=CARTESIAN_POINT('Origin',(-427.260853379936,158.160697256591,-60.2850395075904)) ;
#3420=CARTESIAN_POINT('',(-426.29118891266,160.387769183321,-56.8276944586541)) ;
#3421=CARTESIAN_POINT('',(-429.666345167812,155.606684675614,-51.7677651590675)) ;
#3422=CARTESIAN_POINT('',(-427.978767040236,157.997226929469,-54.2977298088559)) ;
#3423=CARTESIAN_POINT('',(-426.471899935753,158.770260077133,-64.3910496103614)) ;
#3424=CARTESIAN_POINT('',(-426.381544424206,159.579014630227,-60.6093720345077)) ;
#3425=CARTESIAN_POINT('',(-430.027767213998,152.371666463237,-66.8944754624821)) ;
#3426=CARTESIAN_POINT('',(-428.249833574876,155.570963270184,-65.6427625364266)) ;
#3427=CARTESIAN_POINT('',(-433.40292346915,147.590581955531,-61.8345461628956)) ;
#3428=CARTESIAN_POINT('',(-431.715345341574,149.981124209383,-64.3645108126938)) ;
#3429=CARTESIAN_POINT('',(-433.222212446057,149.208091061719,-54.2711910111883)) ;
#3430=CARTESIAN_POINT('',(-433.312567957603,148.399336508625,-58.0528685870419)) ;
#3431=CARTESIAN_POINT('',(-431.444278806934,152.407387868668,-53.019478085123)) ;
#3432=CARTESIAN_POINT('',(-431.927853123794,151.01908136232,-56.341333608517)) ;
#3433=CARTESIAN_POINT('Origin',(-429.847056190905,153.989175569426,-59.3311203107748)) ;
#3434=CARTESIAN_POINT('Origin',(-420.483251253884,155.19941040057,-63.7704695973542)) ;
#3435=CARTESIAN_POINT('',(-423.296864571725,158.602344345039,-56.5174044521504)) ;
#3436=CARTESIAN_POINT('',(-423.477575594818,156.984835238851,-64.0807596038578)) ;
#3437=CARTESIAN_POINT('',(-424.219383064324,158.512786394731,-59.4101157634537)) ;
#3438=CARTESIAN_POINT('',(-422.50834058379,157.492543629999,-59.2328071883088)) ;
#3439=CARTESIAN_POINT('Origin',(-423.363861824057,158.002665012365,-59.3214614758812)) ;
#3440=CARTESIAN_POINT('',(-424.266099582754,158.094635953892,-61.3653568676994)) ;
#3441=CARTESIAN_POINT('',(-424.242741323539,158.303711174311,-60.3877363155766)) ;
#3442=CARTESIAN_POINT('',(-422.55505710222,157.074393189159,-61.1880482925545)) ;
#3443=CARTESIAN_POINT('Origin',(-423.410578342487,157.584514571526,-61.276702580127)) ;
#3444=CARTESIAN_POINT('',(-422.531698843005,157.283468409579,-60.2104277404316)) ;
#3445=CARTESIAN_POINT('Origin',(-423.669198623584,157.167362402809,-61.1813106604454)) ;
#3446=CARTESIAN_POINT('',(-423.072297664414,156.240088851726,-60.9972644531914)) ;
#3447=CARTESIAN_POINT('',(-422.813677383317,156.657241020443,-61.092656372873)) ;
#3448=CARTESIAN_POINT('',(-424.783340144948,157.260331616459,-61.1745730283363)) ;
#3449=CARTESIAN_POINT('',(-424.524719863851,157.677483785175,-61.2699649480179)) ;
#3450=CARTESIAN_POINT('Origin',(-423.927818904681,156.750210234093,-61.0859187407639)) ;
#3451=CARTESIAN_POINT('Origin',(-422.55505710222,157.074393189159,-61.1880482925545)) ;
#3452=CARTESIAN_POINT('',(-423.025581145983,156.658239292566,-59.0420233489456)) ;
#3453=CARTESIAN_POINT('',(-422.766960864886,157.075391461282,-59.1374152686272)) ;
#3454=CARTESIAN_POINT('',(-423.048939405199,156.449164072146,-60.0196439010685)) ;
#3455=CARTESIAN_POINT('Origin',(-424.219383064324,158.512786394731,-59.4101157634537)) ;
#3456=CARTESIAN_POINT('',(-424.736623626517,157.678482057298,-59.2193319240906)) ;
#3457=CARTESIAN_POINT('',(-424.47800334542,158.095634226015,-59.3147238437721)) ;
#3458=CARTESIAN_POINT('',(-424.759981885733,157.469406836878,-60.1969524762134)) ;
#3459=CARTESIAN_POINT('Origin',(-420.910136304531,155.173860616231,-59.7980081821374)) ;
#3460=CARTESIAN_POINT('Origin',(-423.88110238625,157.168360674932,-59.1306776365181)) ;
#3461=CARTESIAN_POINT('Origin',(-423.622482105153,157.585512843649,-59.2260695561997)) ;
#3462=CARTESIAN_POINT('Origin',(-424.039118532129,148.800816786675,-66.2738954494749)) ;
#3463=CARTESIAN_POINT('',(-427.033442873063,150.586241624956,-66.5841854559785)) ;
#3464=CARTESIAN_POINT('',(-426.570653070541,153.468593453358,-65.7447134420378)) ;
#3465=CARTESIAN_POINT('',(-425.651407877875,155.122726175179,-65.0975401929532)) ;
#3466=CARTESIAN_POINT('',(-426.111030474208,154.295659814269,-65.4211268174955)) ;
#3467=CARTESIAN_POINT('',(-424.859610590007,152.448350688626,-65.5674048668929)) ;
#3468=CARTESIAN_POINT('Origin',(-425.715131830274,152.958472070992,-65.6560591544653)) ;
#3469=CARTESIAN_POINT('',(-423.940365397341,154.102483410447,-64.9202316178083)) ;
#3470=CARTESIAN_POINT('',(-424.399987993674,153.275417049536,-65.2438182423506)) ;
#3471=CARTESIAN_POINT('Origin',(-424.795886637608,154.612604792813,-65.0088859053807)) ;
#3472=CARTESIAN_POINT('Origin',(-420.302540230791,156.816919506758,-56.2071144456468)) ;
#3473=CARTESIAN_POINT('',(-426.672020826877,153.821259837333,-51.4574751525639)) ;
#3474=CARTESIAN_POINT('',(-425.403699602451,157.339914614044,-54.7301280175053)) ;
#3475=CARTESIAN_POINT('',(-426.276228276686,156.103932333062,-53.4220601623442)) ;
#3476=CARTESIAN_POINT('',(-425.839963939568,156.721923473553,-54.0760940899247)) ;
#3477=CARTESIAN_POINT('',(-423.692657121916,156.319671849312,-54.5528194423604)) ;
#3478=CARTESIAN_POINT('Origin',(-424.548178362183,156.829793231678,-54.6414737299329)) ;
#3479=CARTESIAN_POINT('',(-424.565185796152,155.08368956833,-53.2447515871992)) ;
#3480=CARTESIAN_POINT('',(-424.128921459034,155.701680708821,-53.8987855147798)) ;
#3481=CARTESIAN_POINT('Origin',(-425.420707036419,155.593810950696,-53.3334058747717)) ;
#3482=CARTESIAN_POINT('Origin',(-427.414274787281,144.019732278968,-61.2139661498883)) ;
#3483=CARTESIAN_POINT('',(-430.408599128215,145.805157117249,-61.524256156392)) ;
#3484=CARTESIAN_POINT('',(-430.012806578024,148.087829612977,-63.488841166182)) ;
#3485=CARTESIAN_POINT('',(-429.140277903789,149.323811893959,-64.7969090213432)) ;
#3486=CARTESIAN_POINT('',(-429.576542240906,148.705820753468,-64.1428750937626)) ;
#3487=CARTESIAN_POINT('',(-428.30176409749,147.067586848245,-63.3115325910371)) ;
#3488=CARTESIAN_POINT('Origin',(-429.157285337757,147.577708230611,-63.4001868786096)) ;
#3489=CARTESIAN_POINT('',(-427.429235423255,148.303569129226,-64.6196004461983)) ;
#3490=CARTESIAN_POINT('',(-427.865499760372,147.685577988735,-63.9655665186177)) ;
#3491=CARTESIAN_POINT('Origin',(-428.284756663522,148.813690511593,-64.7082547337707)) ;
#3492=CARTESIAN_POINT('Origin',(-423.677696485943,152.035834999051,-51.1471851460603)) ;
#3493=CARTESIAN_POINT('',(-430.227888105122,147.422666223438,-53.9609010046846)) ;
#3494=CARTESIAN_POINT('',(-428.845853109934,151.959150773663,-52.4742557416495)) ;
#3495=CARTESIAN_POINT('',(-429.765098302599,150.305018051842,-53.1214289907341)) ;
#3496=CARTESIAN_POINT('',(-429.305475706267,151.132084412752,-52.7978423661918)) ;
#3497=CARTESIAN_POINT('',(-427.1348106294,150.938908008931,-52.2969471665046)) ;
#3498=CARTESIAN_POINT('Origin',(-427.990331869667,151.449029391297,-52.3856014540771)) ;
#3499=CARTESIAN_POINT('',(-428.054055822065,149.284775287109,-52.9441204155892)) ;
#3500=CARTESIAN_POINT('',(-427.594433225732,150.11184164802,-52.6205337910469)) ;
#3501=CARTESIAN_POINT('Origin',(-428.909577062332,149.794896669476,-53.0327747031617)) ;
#3502=CARTESIAN_POINT('Origin',(-427.233563764187,145.637241385156,-53.650610998181)) ;
#3503=CARTESIAN_POINT('',(-431.15040659772,147.333108273129,-56.8536123159879)) ;
#3504=CARTESIAN_POINT('',(-431.197123116151,146.91495783229,-58.8088534202336)) ;
#3505=CARTESIAN_POINT('',(-431.173764856936,147.12403305271,-57.8312328681108)) ;
#3506=CARTESIAN_POINT('',(-429.439364117186,146.312865508397,-56.676303740843)) ;
#3507=CARTESIAN_POINT('Origin',(-430.294885357453,146.822986890763,-56.7649580284154)) ;
#3508=CARTESIAN_POINT('',(-429.486080635617,145.894715067558,-58.6315448450887)) ;
#3509=CARTESIAN_POINT('',(-429.462722376402,146.103790287977,-57.6539242929658)) ;
#3510=CARTESIAN_POINT('Origin',(-430.341601875884,146.404836449924,-58.7201991326612)) ;
#3511=CARTESIAN_POINT('Origin',(-430.036265076356,147.24013905948,-56.860349948097)) ;
#3512=CARTESIAN_POINT('',(-428.922123554992,147.14716984583,-56.8670875802061)) ;
#3513=CARTESIAN_POINT('',(-429.180743836089,146.730017677113,-56.7716956605245)) ;
#3514=CARTESIAN_POINT('',(-430.633166035527,148.167412610562,-57.044396155351)) ;
#3515=CARTESIAN_POINT('',(-430.891786316623,147.750260441846,-56.9490042356694)) ;
#3516=CARTESIAN_POINT('Origin',(-429.77764479526,147.657291228196,-56.9557418677785)) ;
#3517=CARTESIAN_POINT('Origin',(-422.55505710222,157.074393189159,-61.1880482925545)) ;
#3518=CARTESIAN_POINT('',(-428.968840073423,146.729019404991,-58.8223286844518)) ;
#3519=CARTESIAN_POINT('',(-429.22746035452,146.311867236274,-58.7269367647703)) ;
#3520=CARTESIAN_POINT('',(-428.945481814208,146.93809462541,-57.844708132329)) ;
#3521=CARTESIAN_POINT('Origin',(-424.219383064324,158.512786394731,-59.4101157634537)) ;
#3522=CARTESIAN_POINT('',(-430.679882553957,147.749262169723,-58.9996372595968)) ;
#3523=CARTESIAN_POINT('',(-430.938502835054,147.332110001006,-58.9042453399152)) ;
#3524=CARTESIAN_POINT('',(-430.656524294742,147.958337390143,-58.0220167074739)) ;
#3525=CARTESIAN_POINT('Origin',(-426.80667871354,145.662791169495,-57.6230724133978)) ;
#3526=CARTESIAN_POINT('Origin',(-429.82436131369,147.239140787357,-58.9109829720243)) ;
#3527=CARTESIAN_POINT('Origin',(-430.082981594787,146.82198861864,-58.8155910523427)) ;
#3528=CARTESIAN_POINT('Origin',(-424.687602925666,156.530684921226,-55.0170998867998)) ;
#3529=CARTESIAN_POINT('',(-423.971506248882,155.721455228409,-55.3040717560845)) ;
#3530=CARTESIAN_POINT('',(-423.832081685399,156.020563538859,-54.9284455992273)) ;
#3531=CARTESIAN_POINT('',(-425.682548729416,156.741697993141,-55.4813803312294)) ;
#3532=CARTESIAN_POINT('',(-425.543124165933,157.040806303592,-55.1057541743722)) ;
#3533=CARTESIAN_POINT('Origin',(-424.827027489149,156.231576610775,-55.3927260436569)) ;
#3534=CARTESIAN_POINT('Origin',(-422.55505710222,157.074393189159,-61.1880482925545)) ;
#3535=CARTESIAN_POINT('',(-424.844034923117,154.485472947427,-53.9960039009233)) ;
#3536=CARTESIAN_POINT('',(-424.704610359635,154.784581257878,-53.6203777440662)) ;
#3537=CARTESIAN_POINT('',(-424.407770586,155.103464087918,-54.6500378285039)) ;
#3538=CARTESIAN_POINT('Origin',(-424.219383064324,158.512786394731,-59.4101157634537)) ;
#3539=CARTESIAN_POINT('',(-426.555077403651,155.505715712159,-54.1733124760682)) ;
#3540=CARTESIAN_POINT('',(-426.415652840169,155.80482402261,-53.7976863192111)) ;
#3541=CARTESIAN_POINT('',(-426.118813066534,156.12370685265,-54.8273464036488)) ;
#3542=CARTESIAN_POINT('Origin',(-422.268967485332,153.828160632003,-54.4284021095727)) ;
#3543=CARTESIAN_POINT('Origin',(-425.699556163384,154.995594329793,-54.0846581884958)) ;
#3544=CARTESIAN_POINT('Origin',(-425.560131599902,155.294702640244,-53.7090320316386)) ;
#3545=CARTESIAN_POINT('Origin',(-429.017860774274,147.876816541063,-63.0245607217426)) ;
#3546=CARTESIAN_POINT('',(-428.022914970524,147.665803469147,-62.560280277313)) ;
#3547=CARTESIAN_POINT('',(-428.162339534007,147.366695158697,-62.9359064341702)) ;
#3548=CARTESIAN_POINT('',(-429.733957451058,148.68604623388,-62.737588852458)) ;
#3549=CARTESIAN_POINT('',(-429.873382014541,148.386937923429,-63.1132150093151)) ;
#3550=CARTESIAN_POINT('Origin',(-428.878436210791,148.175924851514,-62.6489345648855)) ;
#3551=CARTESIAN_POINT('Origin',(-422.55505710222,157.074393189159,-61.1880482925545)) ;
#3552=CARTESIAN_POINT('',(-427.150386296289,148.901785750129,-63.8683481324742)) ;
#3553=CARTESIAN_POINT('',(-427.289810859772,148.602677439679,-64.2439742893313)) ;
#3554=CARTESIAN_POINT('',(-427.586650633407,148.283794609638,-63.2143142048936)) ;
#3555=CARTESIAN_POINT('Origin',(-424.219383064324,158.512786394731,-59.4101157634537)) ;
#3556=CARTESIAN_POINT('',(-428.861428776823,149.922028514862,-64.0456567076191)) ;
#3557=CARTESIAN_POINT('',(-429.000853340306,149.622920204411,-64.4212828644763)) ;
#3558=CARTESIAN_POINT('',(-429.297693113941,149.304037374371,-63.3916227800385)) ;
#3559=CARTESIAN_POINT('Origin',(-425.447847532739,147.008491153723,-62.9926784859625)) ;
#3560=CARTESIAN_POINT('Origin',(-428.005907536556,149.411907132495,-63.9570024200467)) ;
#3561=CARTESIAN_POINT('Origin',(-428.145332100039,149.112798822045,-64.3326285769038)) ;
#3562=CARTESIAN_POINT('Origin',(-425.834327547888,152.840428212728,-65.1850410779168)) ;
#3563=CARTESIAN_POINT('',(-425.098002025235,152.212262972096,-64.6253687138057)) ;
#3564=CARTESIAN_POINT('',(-424.978806307621,152.330306830362,-65.0963867903444)) ;
#3565=CARTESIAN_POINT('',(-426.809044505769,153.232505736828,-64.8026772889506)) ;
#3566=CARTESIAN_POINT('',(-426.689848788155,153.350549595094,-65.2736953654893)) ;
#3567=CARTESIAN_POINT('Origin',(-425.953523265502,152.722384354462,-64.7140230013782)) ;
#3568=CARTESIAN_POINT('Origin',(-422.55505710222,157.074393189159,-61.1880482925545)) ;
#3569=CARTESIAN_POINT('',(-424.178756832569,153.866395693917,-63.9781954647211)) ;
#3570=CARTESIAN_POINT('',(-424.059561114955,153.984439552183,-64.4492135412598)) ;
#3571=CARTESIAN_POINT('',(-424.638379428902,153.039329333006,-64.3017820892634)) ;
#3572=CARTESIAN_POINT('Origin',(-424.219383064324,158.512786394731,-59.4101157634537)) ;
#3573=CARTESIAN_POINT('',(-425.889799313103,154.886638458649,-64.155504039866)) ;
#3574=CARTESIAN_POINT('',(-425.770603595489,155.004682316915,-64.6265221164047)) ;
#3575=CARTESIAN_POINT('',(-426.349421909436,154.059572097739,-64.4790906644083)) ;
#3576=CARTESIAN_POINT('Origin',(-422.499576328234,151.764025877091,-64.0801463703322)) ;
#3577=CARTESIAN_POINT('Origin',(-425.034278072836,154.376517076283,-64.0668497522936)) ;
#3578=CARTESIAN_POINT('Origin',(-424.915082355222,154.494560934549,-64.5378678288323)) ;
#3579=CARTESIAN_POINT('Origin',(-427.871136152053,151.567073249561,-52.8566195306256)) ;
#3580=CARTESIAN_POINT('',(-426.896419194171,151.174995725461,-53.2389833195918)) ;
#3581=CARTESIAN_POINT('',(-427.015614911786,151.056951867195,-52.7679652430531)) ;
#3582=CARTESIAN_POINT('',(-428.607461674705,152.195238490193,-53.4162918947367)) ;
#3583=CARTESIAN_POINT('',(-428.72665739232,152.077194631927,-52.945273818198)) ;
#3584=CARTESIAN_POINT('Origin',(-427.751940434438,151.685117107827,-53.3276376071643)) ;
#3585=CARTESIAN_POINT('Origin',(-422.55505710222,157.074393189159,-61.1880482925545)) ;
#3586=CARTESIAN_POINT('',(-427.815664386837,149.520863003639,-53.8861565686764)) ;
#3587=CARTESIAN_POINT('',(-427.934860104451,149.402819145373,-53.4151384921377)) ;
#3588=CARTESIAN_POINT('',(-427.356041790504,150.34792936455,-53.5625699441341)) ;
#3589=CARTESIAN_POINT('Origin',(-424.219383064324,158.512786394731,-59.4101157634537)) ;
#3590=CARTESIAN_POINT('',(-429.526706867371,150.541105768372,-54.0634651438213)) ;
#3591=CARTESIAN_POINT('',(-429.645902584985,150.423061910106,-53.5924470672826)) ;
#3592=CARTESIAN_POINT('',(-429.067084271038,151.368172129282,-53.739878519279)) ;
#3593=CARTESIAN_POINT('Origin',(-425.217238689837,149.072625908635,-53.3409342252029)) ;
#3594=CARTESIAN_POINT('Origin',(-428.671185627104,150.030984386006,-53.9748108562489)) ;
#3595=CARTESIAN_POINT('Origin',(-428.790381344718,149.91294052774,-53.5037927797102)) ;
#3596=CARTESIAN_POINT('Origin',(-434.570539808047,161.49079441183,-60.8225683527433)) ;
#3597=CARTESIAN_POINT('',(-433.741264095171,162.693309250613,-61.9058149407666)) ;
#3598=CARTESIAN_POINT('Origin',(-436.691226113041,158.070146628355,-60.0403546113545)) ;
#3599=CARTESIAN_POINT('Origin',(-436.434569740961,157.917110213645,-60.0137583250828)) ;
#3600=CARTESIAN_POINT('',(-433.433353664221,162.818524604835,-61.9789632008915)) ;
#3601=CARTESIAN_POINT('Origin',(-433.484607723091,162.540272835903,-61.8792186544949)) ;
#3602=CARTESIAN_POINT('',(-439.214726609873,154.133897479889,-56.1600302115885)) ;
#3603=CARTESIAN_POINT('Origin',(-436.52605577973,157.97166056537,-60.0232386619911)) ;
#3604=CARTESIAN_POINT('Origin',(-436.52605577973,157.97166056537,-60.0232386619911)) ;
#3605=CARTESIAN_POINT('Origin',(-426.211090919796,151.821159694385,-58.9543395885945)) ;
#3606=CARTESIAN_POINT('',(-428.175935754834,158.45348503928,-59.7105799665025)) ;
#3607=CARTESIAN_POINT('',(-432.681825203754,151.468652058629,-56.4194647576367)) ;
#3608=CARTESIAN_POINT('Origin',(-430.601028270865,154.438746265736,-59.4092514598946)) ;
#3609=CARTESIAN_POINT('',(-428.291887852685,148.851065487279,-55.9645528863367)) ;
#3610=CARTESIAN_POINT('Origin',(-430.601028270865,154.438746265736,-59.4092514598946)) ;
#3611=CARTESIAN_POINT('Origin',(-434.543858272972,156.789736277955,-59.8178313623023)) ;
#3612=CARTESIAN_POINT('',(-432.890930981183,151.522189137641,-56.3869745462188)) ;
#3613=CARTESIAN_POINT('Origin',(-434.543858272972,156.789736277955,-59.8178313623023)) ;
#3614=CARTESIAN_POINT('',(-428.308909482746,158.625038695568,-59.7336968330844)) ;
#3615=CARTESIAN_POINT('Origin',(-430.774976653306,154.542466413331,-59.4272770438238)) ;
#3616=CARTESIAN_POINT('Origin',(-430.774976653306,154.542466413331,-59.4272770438238)) ;
#3617=CARTESIAN_POINT('Origin',(-430.601028270865,154.438746265736,-59.4092514598946)) ;
#3618=CARTESIAN_POINT('Origin',(-428.021142615512,158.709744960995,-59.7298137009669)) ;
#4295=UNCERTAINTY_MEASURE_WITH_UNIT(LENGTH_MEASURE(0.01),#4305,
'DISTANCE_ACCURACY_VALUE',
'Maximum model space distance between geometric entities at asserted c
onnectivities') ;
#4298=UNCERTAINTY_MEASURE_WITH_UNIT(LENGTH_MEASURE(0.01),#4305,
'DISTANCE_ACCURACY_VALUE',
'Maximum model space distance between geometric entities at asserted c
onnectivities') ;
#4301=(
GEOMETRIC_REPRESENTATION_CONTEXT(3)
GLOBAL_UNCERTAINTY_ASSIGNED_CONTEXT((#4295))
GLOBAL_UNIT_ASSIGNED_CONTEXT((#4305,#4307,#4308))
REPRESENTATION_CONTEXT('','3D')
) ;
#4304=(
GEOMETRIC_REPRESENTATION_CONTEXT(3)
GLOBAL_UNCERTAINTY_ASSIGNED_CONTEXT((#4298))
GLOBAL_UNIT_ASSIGNED_CONTEXT((#4305,#4307,#4308))
REPRESENTATION_CONTEXT('','3D')
) ;
#4305=(
LENGTH_UNIT()
NAMED_UNIT(*)
SI_UNIT(.MILLI.,.METRE.)
) ;
#4307=(
NAMED_UNIT(*)
PLANE_ANGLE_UNIT()
SI_UNIT($,.RADIAN.)
) ;
#4308=(
NAMED_UNIT(*)
SI_UNIT($,.STERADIAN.)
SOLID_ANGLE_UNIT()
) ;
#4311=SHAPE_DEFINITION_REPRESENTATION(#4316,#4332) ;
#4316=PRODUCT_DEFINITION_SHAPE('',$,#4338) ;
#4332=SHAPE_REPRESENTATION('',(#2268),#4301) ;
#4335=PRODUCT_DEFINITION_CONTEXT('part definition',#4352,'design') ;
#4338=PRODUCT_DEFINITION('Connector_1-8','Connector_1-8',#4343,#4335) ;
#4343=PRODUCT_DEFINITION_FORMATION('',$,#4356) ;
#4352=APPLICATION_CONTEXT(
'Core Data for Automotive Mechanical Design Process') ;
#4353=PRODUCT_CONTEXT('part definition',#4352,'mechanical') ;
#4356=PRODUCT('Connector_1-8','Connector_1-8',$,(#4353)) ;
#4360=PRESENTATION_STYLE_ASSIGNMENT((#4364)) ;
#4364=SURFACE_STYLE_USAGE(.BOTH.,#4368) ;
#4368=SURFACE_SIDE_STYLE('',(#4372)) ;
#4372=SURFACE_STYLE_FILL_AREA(#4376) ;
#4376=FILL_AREA_STYLE('Opaque(243,203,124)',(#4380)) ;
#4380=FILL_AREA_STYLE_COLOUR('Opaque(243,203,124)',#4384) ;
#4384=COLOUR_RGB('Opaque(243,203,124)', 0.09019608, 0.27058824, 0.51372549) ;
ENDSEC;
END-ISO-10303-21;
